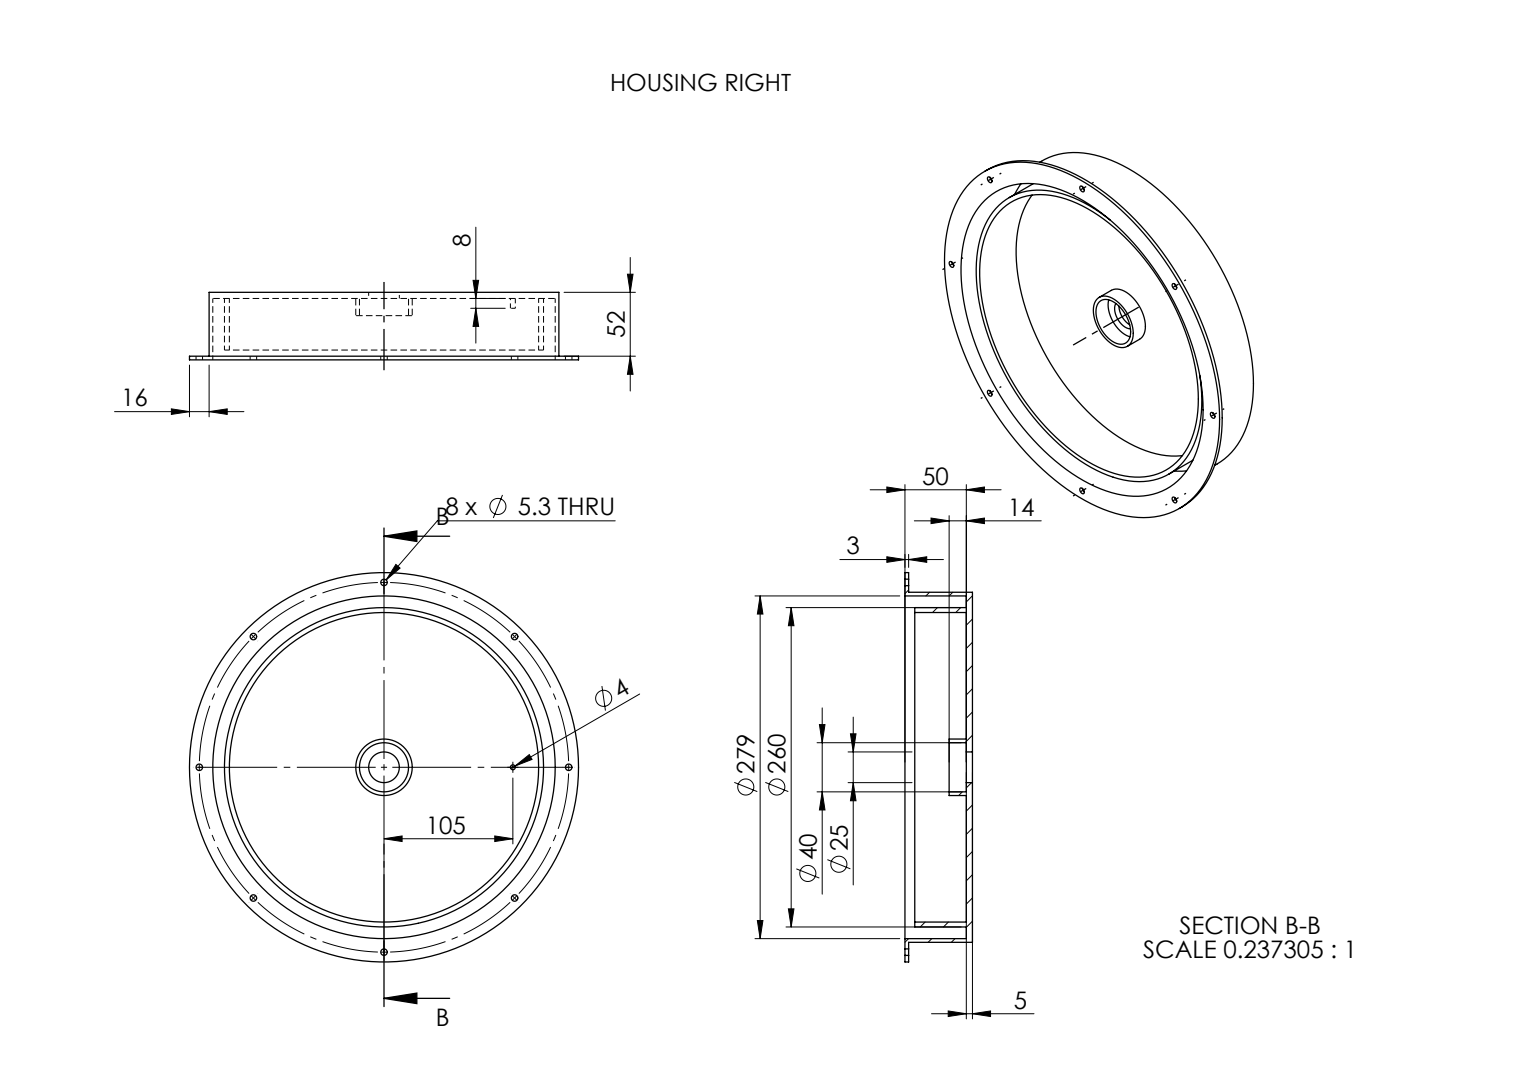
ISO-10303-21;
HEADER;
FILE_DESCRIPTION (('STEP AP214'),
    '1' );
FILE_NAME ('housing right.step',
    '2026-10-08T11:45:07',
    ( '' ),
    ( '' ),
    'SwSTEP 2.0',
    'SolidWorks 2026',
    '' );
FILE_SCHEMA (( 'AUTOMOTIVE_DESIGN' ));
ENDSEC;

DATA;
#35=CIRCLE ( 'NONE', #41130, 12.49999999999993427 ) ;
#48=DIRECTION ( 'NONE',  ( 3.892440008040322386E-16, -2.658563593772947863E-15, -1.000000000000000000 ) ) ;
#71=ORIENTED_EDGE ( 'NONE', *, *, #29230, .F. ) ;
#74=CARTESIAN_POINT ( 'NONE',  ( -3.996523416598931009E-15, 2.658563593772952281E-14, 10.00000000000000178 ) ) ;
#130=EDGE_CURVE ( 'NONE', #29194, #21952, #31734, .T. ) ;
#132=CIRCLE ( 'NONE', #17653, 142.4999999999992610 ) ;
#196=DIRECTION ( 'NONE',  ( -3.996523416598930318E-16, 2.658563593772947863E-15, 1.000000000000000000 ) ) ;
#215=DIRECTION ( 'NONE',  ( 1.000000000000000000, 0.000000000000000000, -3.273063162220425331E-16 ) ) ;
#239=VERTEX_POINT ( 'NONE', #9633 ) ;
#246=CARTESIAN_POINT ( 'NONE',  ( 150.4999999999986926, 1.388241670201576064E-12, 6.999999999999959144 ) ) ;
#281=CARTESIAN_POINT ( 'NONE',  ( 106.9999999999993179, -2.318365118890836037E-13, -32.00000000000000000 ) ) ;
#401=EDGE_CURVE ( 'NONE', #35963, #19047, #6638, .T. ) ;
#561=CIRCLE ( 'NONE', #25023, 12.49999999999993427 ) ;
#699=ORIENTED_EDGE ( 'NONE', *, *, #10056, .T. ) ;
#888=DIRECTION ( 'NONE',  ( 1.000000000000000000, -1.373900992973641868E-15, -3.994789077170585140E-16 ) ) ;
#928=EDGE_CURVE ( 'NONE', #37599, #28601, #37468, .T. ) ;
#942=DIRECTION ( 'NONE',  ( -3.996523416598930318E-16, 2.658563593772947863E-15, 1.000000000000000000 ) ) ;
#955=CARTESIAN_POINT ( 'NONE',  ( -139.4999999999992610, 2.182448244575515701E-13, 10.00000000000005684 ) ) ;
#1042=FACE_BOUND ( 'NONE', #4502, .T. ) ;
#1092=EDGE_LOOP ( 'NONE', ( #29241, #12983 ) ) ;
#1130=AXIS2_PLACEMENT_3D ( 'NONE', #36549, #35909, #36340 ) ;
#1195=CARTESIAN_POINT ( 'NONE',  ( -2.107686228591307694E-13, 150.5000000000013642, 10.00000000000041922 ) ) ;
#1201=CIRCLE ( 'NONE', #28408, 158.4999999999992042 ) ;
#1256=DIRECTION ( 'NONE',  ( -3.996523416598930318E-16, 2.658563593772947863E-15, 1.000000000000000000 ) ) ;
#1258=CARTESIAN_POINT ( 'NONE',  ( -106.4195705685749402, 106.4195705685765745, 7.000000000000337508 ) ) ;
#1259=VECTOR ( 'NONE', #5273, 1000.000000000000000 ) ;
#1261=DIRECTION ( 'NONE',  ( -3.996523416598930318E-16, 2.658563593772947863E-15, 1.000000000000000000 ) ) ;
#1275=PLANE ( 'NONE',  #36174 ) ;
#1282=DIRECTION ( 'NONE',  ( 1.000000000000000000, -1.373900992973641868E-15, -3.994789077170585140E-16 ) ) ;
#1310=DIRECTION ( 'NONE',  ( -3.996523416598930318E-16, 2.658563593772947863E-15, 1.000000000000000000 ) ) ;
#1351=ORIENTED_EDGE ( 'NONE', *, *, #21891, .F. ) ;
#1373=FILL_AREA_STYLE ('',( #25619 ) ) ;
#1422=DIRECTION ( 'NONE',  ( 1.000000000000000000, 0.000000000000000000, -6.546126324440832913E-16 ) ) ;
#1454=CIRCLE ( 'NONE', #18933, 2.649999999999979039 ) ;
#1460=AXIS2_PLACEMENT_3D ( 'NONE', #22396, #26282, #32380 ) ;
#1470=DIRECTION ( 'NONE',  ( 1.000000000000000000, 0.000000000000000000, -6.546126324440850663E-16 ) ) ;
#1495=AXIS2_PLACEMENT_3D ( 'NONE', #18764, #1256, #11313 ) ;
#1513=EDGE_CURVE ( 'NONE', #34370, #34755, #40157, .T. ) ;
#1523=DIRECTION ( 'NONE',  ( -3.996523416598930318E-16, 2.658563593772947863E-15, 1.000000000000000000 ) ) ;
#1539=ADVANCED_FACE ( 'NONE', ( #18278 ), #14551, .T. ) ;
#1612=ORIENTED_EDGE ( 'NONE', *, *, #24949, .T. ) ;
#1654=EDGE_CURVE ( 'NONE', #20992, #25205, #27692, .T. ) ;
#1669=VECTOR ( 'NONE', #942, 1000.000000000000000 ) ;
#1692=LINE ( 'NONE', #4529, #37119 ) ;
#1705=EDGE_CURVE ( 'NONE', #13925, #12177, #32177, .T. ) ;
#1804=SURFACE_STYLE_USAGE ( .BOTH. , #18872 ) ;
#1807=EDGE_LOOP ( 'NONE', ( #11294, #17144 ) ) ;
#1888=AXIS2_PLACEMENT_3D ( 'NONE', #35141, #2178, #24725 ) ;
#2004=EDGE_CURVE ( 'NONE', #41484, #24680, #21070, .T. ) ;
#2042=ORIENTED_EDGE ( 'NONE', *, *, #2004, .T. ) ;
#2045=DIRECTION ( 'NONE',  ( 3.996523416598993920E-16, 2.658563593772947074E-15, 1.000000000000000000 ) ) ;
#2057=EDGE_CURVE ( 'NONE', #25205, #20992, #33192, .T. ) ;
#2087=VECTOR ( 'NONE', #14850, 1000.000000000000000 ) ;
#2101=DIRECTION ( 'NONE',  ( -3.996523416598930318E-16, 2.658563593772947863E-15, 1.000000000000000000 ) ) ;
#2138=DIRECTION ( 'NONE',  ( 3.996523416598930318E-16, -2.658563593772947863E-15, -1.000000000000000000 ) ) ;
#2151=VERTEX_POINT ( 'NONE', #41176 ) ;
#2178=DIRECTION ( 'NONE',  ( -3.996523416598930318E-16, 2.658563593772947863E-15, 1.000000000000000000 ) ) ;
#2190=CARTESIAN_POINT ( 'NONE',  ( 104.9999999999993321, -2.506021480131494702E-13, -40.00000000000000000 ) ) ;
#2216=SURFACE_STYLE_USAGE ( .BOTH. , #5718 ) ;
#2237=DIRECTION ( 'NONE',  ( 3.996523416598930318E-16, -2.658563593772947863E-15, -1.000000000000000000 ) ) ;
#2270=ORIENTED_EDGE ( 'NONE', *, *, #38290, .T. ) ;
#2365=CARTESIAN_POINT ( 'NONE',  ( 23.00000000000001066, -1.165156337948621952E-13, -25.99999999999999289 ) ) ;
#2396=ORIENTED_EDGE ( 'NONE', *, *, #28334, .F. ) ;
#2434=PLANE ( 'NONE',  #33908 ) ;
#2445=CARTESIAN_POINT ( 'NONE',  ( -24.83242019125695421, 113.3108596183312216, 2.000000000000327738 ) ) ;
#2465=EDGE_CURVE ( 'NONE', #28601, #37599, #42175, .T. ) ;
#2478=DIRECTION ( 'NONE',  ( -3.996523416598930318E-16, 2.658563593772947863E-15, 1.000000000000000000 ) ) ;
#2537=AXIS2_PLACEMENT_3D ( 'NONE', #41329, #11482, #24817 ) ;
#2636=CYLINDRICAL_SURFACE ( 'NONE', #18326, 158.4999999999992042 ) ;
#2638=EDGE_CURVE ( 'NONE', #38278, #24835, #38702, .T. ) ;
#2665=DIRECTION ( 'NONE',  ( 1.000000000000000000, -1.373900992973642263E-15, 0.000000000000000000 ) ) ;
#2673=CYLINDRICAL_SURFACE ( 'NONE', #25111, 19.99999999999989342 ) ;
#2692=CYLINDRICAL_SURFACE ( 'NONE', #35754, 2.649999999999979039 ) ;
#2714=EDGE_LOOP ( 'NONE', ( #26003, #5036, #29046, #42550 ) ) ;
#2731=CYLINDRICAL_SURFACE ( 'NONE', #26813, 12.49999999999993427 ) ;
#2791=EDGE_CURVE ( 'NONE', #36354, #9697, #17894, .T. ) ;
#2817=DIRECTION ( 'NONE',  ( 1.000000000000000000, 0.000000000000000000, -3.273063162220416457E-16 ) ) ;
#2847=EDGE_LOOP ( 'NONE', ( #27807, #15265 ) ) ;
#2852=CARTESIAN_POINT ( 'NONE',  ( -139.4999999999999716, 1.517807346132291325E-13, -40.00000000000005684 ) ) ;
#2893=DIRECTION ( 'NONE',  ( -3.996523416598930318E-16, 2.658563593772947863E-15, 1.000000000000000000 ) ) ;
#2967=CARTESIAN_POINT ( 'NONE',  ( -142.5000000000000000, 1.627194001049080943E-13, -45.00000000000004974 ) ) ;
#2977=CARTESIAN_POINT ( 'NONE',  ( 126.0000000000000568, -2.077321393419925476E-13, -39.99999999999992895 ) ) ;
#3020=DIRECTION ( 'NONE',  ( -1.000000000000000000, 1.373900992973641868E-15, 3.469446951953632924E-16 ) ) ;
#3024=ADVANCED_FACE ( 'NONE', ( #26080 ), #9700, .F. ) ;
#3066=FACE_BOUND ( 'NONE', #13828, .T. ) ;
#3120=DIRECTION ( 'NONE',  ( -3.996523416598930318E-16, 2.658563593772947863E-15, 1.000000000000000000 ) ) ;
#3131=DIRECTION ( 'NONE',  ( -3.996523416598930318E-16, 2.658563593772947863E-15, 1.000000000000000000 ) ) ;
#3156=CARTESIAN_POINT ( 'NONE',  ( -19.99999999999998934, -6.025457873503454466E-14, -26.00000000000001066 ) ) ;
#3170=AXIS2_PLACEMENT_3D ( 'NONE', #25052, #18077, #31766 ) ;
#3264=AXIS2_PLACEMENT_3D ( 'NONE', #13667, #24140, #3577 ) ;
#3280=EDGE_LOOP ( 'NONE', ( #4077, #12239, #21262, #32611 ) ) ;
#3329=AXIS2_PLACEMENT_3D ( 'NONE', #11939, #28527, #38091 ) ;
#3410=DIRECTION ( 'NONE',  ( 1.000000000000000000, 0.000000000000000000, -6.546126324440850663E-16 ) ) ;
#3459=ADVANCED_FACE ( 'NONE', ( #5721 ), #35603, .F. ) ;
#3474=DIRECTION ( 'NONE',  ( 1.000000000000000000, -1.373900992973641868E-15, -4.017254365419995317E-16 ) ) ;
#3539=DIRECTION ( 'NONE',  ( -3.996523416598930318E-16, 2.658563593772947863E-15, 1.000000000000000000 ) ) ;
#3549=VERTEX_POINT ( 'NONE', #2852 ) ;
#3577=DIRECTION ( 'NONE',  ( 1.000000000000000000, -1.373900992973642066E-15, -3.854941057726257326E-16 ) ) ;
#3634=ADVANCED_FACE ( 'NONE', ( #29950 ), #24291, .F. ) ;
#3638=EDGE_CURVE ( 'NONE', #11569, #32279, #21241, .T. ) ;
#3662=EDGE_LOOP ( 'NONE', ( #38086, #23873 ) ) ;
#3722=CARTESIAN_POINT ( 'NONE',  ( 147.8499999999987153, 1.396194884625391392E-12, 9.999999999999960920 ) ) ;
#3733=AXIS2_PLACEMENT_3D ( 'NONE', #39429, #9127, #6070 ) ;
#3754=ORIENTED_EDGE ( 'NONE', *, *, #35389, .T. ) ;
#3757=ORIENTED_EDGE ( 'NONE', *, *, #35139, .T. ) ;
#3773=ORIENTED_EDGE ( 'NONE', *, *, #30193, .T. ) ;
#3794=ADVANCED_FACE ( 'NONE', ( #21234 ), #31884, .F. ) ;
#3839=EDGE_LOOP ( 'NONE', ( #23186, #13408 ) ) ;
#3852=CARTESIAN_POINT ( 'NONE',  ( 0.000000000000000000, 0.000000000000000000, 0.000000000000000000 ) ) ;
#3970=VECTOR ( 'NONE', #21919, 1000.000000000000000 ) ;
#4011=CARTESIAN_POINT ( 'NONE',  ( 106.4195705685734623, 106.4195705685780524, 10.00000000000025402 ) ) ;
#4044=AXIS2_PLACEMENT_3D ( 'NONE', #5844, #28374, #14845 ) ;
#4077=ORIENTED_EDGE ( 'NONE', *, *, #40367, .F. ) ;
#4086=ADVANCED_FACE ( 'NONE', ( #31583 ), #28757, .F. ) ;
#4136=ORIENTED_EDGE ( 'NONE', *, *, #8514, .T. ) ;
#4160=ADVANCED_BREP_SHAPE_REPRESENTATION ( '', ( #13589, #13552 ), #31631 ) ;
#4180=DIRECTION ( 'NONE',  ( -3.996523416598930318E-16, 2.658563593772947863E-15, 1.000000000000000000 ) ) ;
#4181=EDGE_LOOP ( 'NONE', ( #12378, #30826, #3773, #26628 ) ) ;
#4221=FACE_BOUND ( 'NONE', #10756, .T. ) ;
#4254=ORIENTED_EDGE ( 'NONE', *, *, #1513, .T. ) ;
#4297=DIRECTION ( 'NONE',  ( -3.996523416598930318E-16, 2.658563593772947863E-15, 1.000000000000000000 ) ) ;
#4303=DIRECTION ( 'NONE',  ( -3.996523416598930318E-16, 2.658563593772947863E-15, 1.000000000000000000 ) ) ;
#4332=ORIENTED_EDGE ( 'NONE', *, *, #24391, .F. ) ;
#4344=VERTEX_POINT ( 'NONE', #7599 ) ;
#4367=ORIENTED_EDGE ( 'NONE', *, *, #36129, .F. ) ;
#4368=CARTESIAN_POINT ( 'NONE',  ( -109.0695705685749317, 106.4195705685765603, 10.00000000000033573 ) ) ;
#4438=CARTESIAN_POINT ( 'NONE',  ( 1.598609366639573350E-14, -1.063425437509180407E-13, -40.00000000000000000 ) ) ;
#4449=AXIS2_PLACEMENT_3D ( 'NONE', #40376, #7006, #20157 ) ;
#4454=ORIENTED_EDGE ( 'NONE', *, *, #7875, .F. ) ;
#4488=DIRECTION ( 'NONE',  ( -3.996523416598930318E-16, 2.658563593772947863E-15, 1.000000000000000000 ) ) ;
#4502=EDGE_LOOP ( 'NONE', ( #15982, #4454 ) ) ;
#4513=DIRECTION ( 'NONE',  ( -1.000000000000000000, 1.373900992973642066E-15, 3.979293995072266947E-16 ) ) ;
#4529=CARTESIAN_POINT ( 'NONE',  ( 109.0695705685756565, -106.4195705685758213, 9.999999999999667821 ) ) ;
#4583=EDGE_LOOP ( 'NONE', ( #30063, #12227 ) ) ;
#4597=CARTESIAN_POINT ( 'NONE',  ( -109.0695705685741785, -106.4195705685773135, 6.999999999999753975 ) ) ;
#4724=VECTOR ( 'NONE', #10466, 1000.000000000000000 ) ;
#4732=DIRECTION ( 'NONE',  ( 1.000000000000000000, 0.000000000000000000, -6.546126324440832913E-16 ) ) ;
#4747=DIRECTION ( 'NONE',  ( -3.996523416598930318E-16, 2.658563593772947863E-15, 1.000000000000000000 ) ) ;
#4775=VECTOR ( 'NONE', #27728, 1000.000000000000000 ) ;
#4776=FACE_BOUND ( 'NONE', #41078, .T. ) ;
#4870=( NAMED_UNIT ( * ) SI_UNIT ( $, .STERADIAN. ) SOLID_ANGLE_UNIT ( ) );
#4942=CARTESIAN_POINT ( 'NONE',  ( 1.798435537469519230E-14, -1.196353617197826191E-13, -44.99999999999999289 ) ) ;
#4970=DIRECTION ( 'NONE',  ( 1.000000000000000000, -1.373900992973642066E-15, -3.979293995072266947E-16 ) ) ;
#4973=CIRCLE ( 'NONE', #7043, 2.649999999999973266 ) ;
#5036=ORIENTED_EDGE ( 'NONE', *, *, #1654, .F. ) ;
#5038=DIRECTION ( 'NONE',  ( -3.996523416598930318E-16, 2.658563593772947863E-15, 1.000000000000000000 ) ) ;
#5113=FACE_BOUND ( 'NONE', #4583, .T. ) ;
#5117=VERTEX_POINT ( 'NONE', #25453 ) ;
#5125=DIRECTION ( 'NONE',  ( 1.000000000000000000, 0.000000000000000000, -3.273063162220416457E-16 ) ) ;
#5129=CIRCLE ( 'NONE', #23286, 2.649999999999957723 ) ;
#5147=EDGE_CURVE ( 'NONE', #34755, #34370, #1454, .T. ) ;
#5259=AXIS2_PLACEMENT_3D ( 'NONE', #8434, #21998, #4732 ) ;
#5273=DIRECTION ( 'NONE',  ( -3.996523416598930318E-16, 2.658563593772947863E-15, 1.000000000000000000 ) ) ;
#5304=CIRCLE ( 'NONE', #6656, 125.9999999999993605 ) ;
#5453=AXIS2_PLACEMENT_3D ( 'NONE', #39950, #22798, #39534 ) ;
#5480=CARTESIAN_POINT ( 'NONE',  ( 1.598609366639573350E-14, -1.063425437509180407E-13, -40.00000000000000000 ) ) ;
#5595=CARTESIAN_POINT ( 'NONE',  ( -103.7695705685749772, 106.4195705685765745, 10.00000000000033396 ) ) ;
#5623=ORIENTED_EDGE ( 'NONE', *, *, #10507, .F. ) ;
#5650=AXIS2_PLACEMENT_3D ( 'NONE', #27391, #20437, #13666 ) ;
#5678=ORIENTED_EDGE ( 'NONE', *, *, #24651, .T. ) ;
#5693=ORIENTED_EDGE ( 'NONE', *, *, #25641, .F. ) ;
#5714=DIRECTION ( 'NONE',  ( -3.996523416598930318E-16, 2.658563593772947863E-15, 1.000000000000000000 ) ) ;
#5718=SURFACE_SIDE_STYLE ('',( #38885 ) ) ;
#5721=FACE_OUTER_BOUND ( 'NONE', #3280, .T. ) ;
#5724=ORIENTED_EDGE ( 'NONE', *, *, #35189, .T. ) ;
#5740=ORIENTED_EDGE ( 'NONE', *, *, #21265, .T. ) ;
#5743=CYLINDRICAL_SURFACE ( 'NONE', #28436, 2.649999999999971934 ) ;
#5782=CYLINDRICAL_SURFACE ( 'NONE', #3329, 12.49999999999993427 ) ;
#5803=ORIENTED_EDGE ( 'NONE', *, *, #37006, .T. ) ;
#5818=CIRCLE ( 'NONE', #29501, 19.99999999999989342 ) ;
#5844=CARTESIAN_POINT ( 'NONE',  ( -106.4195705685749402, 106.4195705685765745, 10.00000000000033573 ) ) ;
#5846=AXIS2_PLACEMENT_3D ( 'NONE', #24235, #10672, #33575 ) ;
#5854=ORIENTED_EDGE ( 'NONE', *, *, #928, .T. ) ;
#5921=CARTESIAN_POINT ( 'NONE',  ( 1.039096088315723056E-14, -6.912265343809663812E-14, -26.00000000000000355 ) ) ;
#5922=AXIS2_PLACEMENT_3D ( 'NONE', #1195, #41554, #11702 ) ;
#5942=DIRECTION ( 'NONE',  ( -3.996523416598930318E-16, 2.658563593772947863E-15, 1.000000000000000000 ) ) ;
#5971=AXIS2_PLACEMENT_3D ( 'NONE', #27064, #34441, #1282 ) ;
#6033=DIRECTION ( 'NONE',  ( 1.000000000000000000, -1.373900992973641277E-15, -5.551115123125812284E-16 ) ) ;
#6070=DIRECTION ( 'NONE',  ( 1.000000000000000000, 0.000000000000000000, -3.273063162220425331E-16 ) ) ;
#6101=AXIS2_PLACEMENT_3D ( 'NONE', #2445, #15809, #42388 ) ;
#6122=CIRCLE ( 'NONE', #10304, 19.99999999999989342 ) ;
#6221=CARTESIAN_POINT ( 'NONE',  ( 139.5000000000000284, -2.144538195783110118E-13, -39.99999999999994316 ) ) ;
#6239=DIRECTION ( 'NONE',  ( -3.996523416598930318E-16, 2.658563593772947863E-15, 1.000000000000000000 ) ) ;
#6244=VERTEX_POINT ( 'NONE', #26614 ) ;
#6245=CARTESIAN_POINT ( 'NONE',  ( 1.798435537469519230E-14, -1.196353617197826191E-13, -44.99999999999999289 ) ) ;
#6312=ADVANCED_FACE ( 'NONE', ( #24231, #17911, #20746, #31186, #4776, #30544, #1042, #34655, #27473, #37497 ), #1275, .T. ) ;
#6331=FACE_OUTER_BOUND ( 'NONE', #38808, .T. ) ;
#6413=DIRECTION ( 'NONE',  ( 3.996523416598930318E-16, -2.658563593772947863E-15, -1.000000000000000000 ) ) ;
#6414=CIRCLE ( 'NONE', #30821, 125.9999999999993605 ) ;
#6445=DIRECTION ( 'NONE',  ( -3.996523416598930318E-16, 2.658563593772947863E-15, 1.000000000000000000 ) ) ;
#6505=STYLED_ITEM ( 'NONE', ( #31931 ), #4160 ) ;
#6638=CIRCLE ( 'NONE', #12249, 158.4999999999992042 ) ;
#6650=DIRECTION ( 'NONE',  ( 1.000000000000000000, 0.000000000000000000, -6.546126324440850663E-16 ) ) ;
#6656=AXIS2_PLACEMENT_3D ( 'NONE', #24085, #30618, #37573 ) ;
#6696=ORIENTED_EDGE ( 'NONE', *, *, #33011, .F. ) ;
#6721=AXIS2_PLACEMENT_3D ( 'NONE', #39446, #9352, #9581 ) ;
#6826=CYLINDRICAL_SURFACE ( 'NONE', #23976, 2.649999999999979039 ) ;
#6875=CYLINDRICAL_SURFACE ( 'NONE', #5650, 129.9999999999993463 ) ;
#6926=CARTESIAN_POINT ( 'NONE',  ( -150.4999999999986926, -2.921102061156358310E-13, 10.00000000000004441 ) ) ;
#6938=FACE_OUTER_BOUND ( 'NONE', #28430, .T. ) ;
#6992=DIRECTION ( 'NONE',  ( 1.000000000000000000, 0.000000000000000000, -6.546126324440850663E-16 ) ) ;
#7001=ORIENTED_EDGE ( 'NONE', *, *, #12745, .T. ) ;
#7004=CIRCLE ( 'NONE', #41129, 2.649999999999971934 ) ;
#7006=DIRECTION ( 'NONE',  ( -3.996523416598930318E-16, 2.658563593772947863E-15, 1.000000000000000000 ) ) ;
#7038=ORIENTED_EDGE ( 'NONE', *, *, #33624, .T. ) ;
#7039=AXIS2_PLACEMENT_3D ( 'NONE', #8455, #21605, #15266 ) ;
#7043=AXIS2_PLACEMENT_3D ( 'NONE', #13886, #33052, #27182 ) ;
#7081=DIRECTION ( 'NONE',  ( -3.996523416598930318E-16, 2.658563593772947863E-15, 1.000000000000000000 ) ) ;
#7134=ORIENTED_EDGE ( 'NONE', *, *, #39605, .F. ) ;
#7188=VERTEX_POINT ( 'NONE', #4597 ) ;
#7241=DIRECTION ( 'NONE',  ( 3.996523416598930318E-16, -2.658563593772947863E-15, -1.000000000000000000 ) ) ;
#7243=CARTESIAN_POINT ( 'NONE',  ( -19.99999999999998224, -6.025457873503436795E-14, -40.00000000000000711 ) ) ;
#7277=CARTESIAN_POINT ( 'NONE',  ( 1.598609366639573350E-14, -1.063425437509180407E-13, -40.00000000000000000 ) ) ;
#7296=DIRECTION ( 'NONE',  ( -3.996523416598930318E-16, 2.658563593772947863E-15, 1.000000000000000000 ) ) ;
#7301=ORIENTED_EDGE ( 'NONE', *, *, #40139, .F. ) ;
#7463=EDGE_LOOP ( 'NONE', ( #17351, #12263, #14343, #4367 ) ) ;
#7512=DIRECTION ( 'NONE',  ( 3.996523416598930318E-16, -2.658563593772947863E-15, -1.000000000000000000 ) ) ;
#7517=CARTESIAN_POINT ( 'NONE',  ( -103.7695705685742240, -106.4195705685773135, 9.999999999999751310 ) ) ;
#7578=EDGE_CURVE ( 'NONE', #7188, #43139, #14414, .T. ) ;
#7588=AXIS2_PLACEMENT_3D ( 'NONE', #22582, #15593, #28897 ) ;
#7599=CARTESIAN_POINT ( 'NONE',  ( -126.0000000000000284, 1.230603612181078346E-13, 1.999999999999952704 ) ) ;
#7651=EDGE_CURVE ( 'NONE', #22603, #21952, #28587, .T. ) ;
#7692=CARTESIAN_POINT ( 'NONE',  ( 1.798435537469519230E-14, -1.196353617197826191E-13, -44.99999999999999289 ) ) ;
#7695=CARTESIAN_POINT ( 'NONE',  ( 106.9999999999993321, -2.424707662641753068E-13, -40.00000000000000000 ) ) ;
#7718=ADVANCED_FACE ( 'NONE', ( #31204 ), #41858, .F. ) ;
#7741=DIRECTION ( 'NONE',  ( 1.000000000000000000, -1.373900992973642263E-15, -3.736327486719295592E-16 ) ) ;
#7809=DIRECTION ( 'NONE',  ( -3.996523416598930318E-16, 2.658563593772947863E-15, 1.000000000000000000 ) ) ;
#7818=ORIENTED_EDGE ( 'NONE', *, *, #12311, .T. ) ;
#7836=ORIENTED_EDGE ( 'NONE', *, *, #9323, .F. ) ;
#7875=EDGE_CURVE ( 'NONE', #42975, #29643, #20300, .T. ) ;
#7923=ADVANCED_FACE ( 'NONE', ( #29431, #26156, #25539 ), #39431, .T. ) ;
#7932=ORIENTED_EDGE ( 'NONE', *, *, #19309, .T. ) ;
#7977=CYLINDRICAL_SURFACE ( 'NONE', #13481, 2.649999999999979039 ) ;
#8063=CARTESIAN_POINT ( 'NONE',  ( -109.0695705685749317, 106.4195705685765603, 7.000000000000336620 ) ) ;
#8203=ORIENTED_EDGE ( 'NONE', *, *, #23450, .F. ) ;
#8284=CIRCLE ( 'NONE', #31276, 130.0000000000013927 ) ;
#8285=ORIENTED_EDGE ( 'NONE', *, *, #26316, .F. ) ;
#8329=ORIENTED_EDGE ( 'NONE', *, *, #35389, .F. ) ;
#8423=ADVANCED_FACE ( 'NONE', ( #17167 ), #6875, .T. ) ;
#8434=CARTESIAN_POINT ( 'NONE',  ( 2.027755760259328333E-13, -150.5000000000013642, 9.999999999999586109 ) ) ;
#8455=CARTESIAN_POINT ( 'NONE',  ( 104.9999999999993321, -2.293336392629658115E-13, -32.00000000000000000 ) ) ;
#8514=EDGE_CURVE ( 'NONE', #21952, #29194, #4973, .T. ) ;
#8531=DIRECTION ( 'NONE',  ( 1.000000000000000000, -1.373900992973642066E-15, -3.854941057726257326E-16 ) ) ;
#8539=EDGE_LOOP ( 'NONE', ( #27289, #22347, #21596, #18498 ) ) ;
#8607=EDGE_CURVE ( 'NONE', #29204, #43139, #14059, .T. ) ;
#8658=DIRECTION ( 'NONE',  ( 3.996523416598930318E-16, -2.658563593772947863E-15, -1.000000000000000000 ) ) ;
#8698=CARTESIAN_POINT ( 'NONE',  ( 2.649999999999768541, 150.5000000000013642, 10.00000000000041567 ) ) ;
#8724=VERTEX_POINT ( 'NONE', #19900 ) ;
#8768=VECTOR ( 'NONE', #2893, 1000.000000000000000 ) ;
#8786=( NAMED_UNIT ( * ) PLANE_ANGLE_UNIT ( ) SI_UNIT ( $, .RADIAN. ) );
#8921=FACE_OUTER_BOUND ( 'NONE', #36499, .T. ) ;
#9017=CARTESIAN_POINT ( 'NONE',  ( 1.598609366639573350E-14, -1.063425437509180407E-13, -40.00000000000000000 ) ) ;
#9023=PLANE ( 'NONE',  #6101 ) ;
#9026=SHAPE_REPRESENTATION ( 'housing right', ( #13552 ), #31631 ) ;
#9076=CARTESIAN_POINT ( 'NONE',  ( 2.649999999999769873, 150.5000000000013642, 7.000000000000418332 ) ) ;
#9088=CARTESIAN_POINT ( 'NONE',  ( 129.9999999999992042, 8.206338904687194424E-13, 369.6955262170047263 ) ) ;
#9127=DIRECTION ( 'NONE',  ( -3.996523416598930318E-16, 2.658563593772947863E-15, 1.000000000000000000 ) ) ;
#9132=LINE ( 'NONE', #15708, #23630 ) ;
#9154=VERTEX_POINT ( 'NONE', #8063 ) ;
#9219=ORIENTED_EDGE ( 'NONE', *, *, #20013, .T. ) ;
#9323=EDGE_CURVE ( 'NONE', #37475, #5117, #132, .T. ) ;
#9352=DIRECTION ( 'NONE',  ( 3.996523416598930318E-16, -2.658563593772947863E-15, -1.000000000000000000 ) ) ;
#9359=ORIENTED_EDGE ( 'NONE', *, *, #31108, .F. ) ;
#9525=ORIENTED_EDGE ( 'NONE', *, *, #1654, .T. ) ;
#9565=ORIENTED_EDGE ( 'NONE', *, *, #20142, .F. ) ;
#9581=DIRECTION ( 'NONE',  ( -1.000000000000000000, 1.373900992973642066E-15, 4.525365589504737954E-16 ) ) ;
#9604=ORIENTED_EDGE ( 'NONE', *, *, #33858, .F. ) ;
#9633=CARTESIAN_POINT ( 'NONE',  ( 130.0000000000000568, -2.127378845942283338E-13, -39.99999999999995026 ) ) ;
#9681=ORIENTED_EDGE ( 'NONE', *, *, #26998, .F. ) ;
#9697=VERTEX_POINT ( 'NONE', #16524 ) ;
#9700=CYLINDRICAL_SURFACE ( 'NONE', #12217, 125.9999999999993605 ) ;
#9745=ORIENTED_EDGE ( 'NONE', *, *, #3638, .T. ) ;
#9749=EDGE_CURVE ( 'NONE', #26054, #42401, #12804, .T. ) ;
#9767=EDGE_CURVE ( 'NONE', #34370, #21317, #15659, .T. ) ;
#9776=CYLINDRICAL_SURFACE ( 'NONE', #37511, 2.649999999999957723 ) ;
#9828=EDGE_CURVE ( 'NONE', #9154, #6244, #26524, .T. ) ;
#9831=CARTESIAN_POINT ( 'NONE',  ( 142.4999999999992610, -1.771709463423323217E-13, 6.999999999999945821 ) ) ;
#9873=VECTOR ( 'NONE', #33300, 1000.000000000000000 ) ;
#9919=CYLINDRICAL_SURFACE ( 'NONE', #41503, 158.4999999999992042 ) ;
#10056=EDGE_CURVE ( 'NONE', #22786, #24835, #17828, .T. ) ;
#10082=DIRECTION ( 'NONE',  ( -3.996523416598930318E-16, 2.658563593772947863E-15, 1.000000000000000000 ) ) ;
#10133=AXIS2_PLACEMENT_3D ( 'NONE', #35928, #42902, #42262 ) ;
#10137=DIRECTION ( 'NONE',  ( 1.000000000000000000, -1.373900992973641868E-15, -4.049512215214018063E-16 ) ) ;
#10148=CARTESIAN_POINT ( 'NONE',  ( 103.7695705685734850, 106.4195705685780524, 10.00000000000025402 ) ) ;
#10213=DIRECTION ( 'NONE',  ( 1.000000000000000000, 0.000000000000000000, 0.000000000000000000 ) ) ;
#10245=VECTOR ( 'NONE', #3131, 1000.000000000000000 ) ;
#10271=AXIS2_PLACEMENT_3D ( 'NONE', #31318, #31742, #24801 ) ;
#10276=AXIS2_PLACEMENT_3D ( 'NONE', #15594, #2237, #26264 ) ;
#10304=AXIS2_PLACEMENT_3D ( 'NONE', #4438, #30868, #37610 ) ;
#10347=ORIENTED_EDGE ( 'NONE', *, *, #33012, .T. ) ;
#10381=CARTESIAN_POINT ( 'NONE',  ( -106.4195705685749402, 106.4195705685765745, 7.000000000000337508 ) ) ;
#10387=CARTESIAN_POINT ( 'NONE',  ( 22.99999999999988987, -9.790568863845134872E-14, -26.00000000000001421 ) ) ;
#10412=DIRECTION ( 'NONE',  ( -3.996523416598930318E-16, 2.658563593772947863E-15, 1.000000000000000000 ) ) ;
#10466=DIRECTION ( 'NONE',  ( 3.996523416598930318E-16, -2.658563593772947863E-15, -1.000000000000000000 ) ) ;
#10471=ORIENTED_EDGE ( 'NONE', *, *, #33011, .T. ) ;
#10486=ORIENTED_EDGE ( 'NONE', *, *, #32018, .F. ) ;
#10492=CARTESIAN_POINT ( 'NONE',  ( -2.797566391619251075E-15, 1.860994515641065082E-14, 7.000000000000002665 ) ) ;
#10507=EDGE_CURVE ( 'NONE', #26054, #25656, #35, .T. ) ;
#10510=AXIS2_PLACEMENT_3D ( 'NONE', #25918, #12398, #4970 ) ;
#10571=CIRCLE ( 'NONE', #1495, 19.99999999999989342 ) ;
#10572=EDGE_LOOP ( 'NONE', ( #20458, #14340 ) ) ;
#10596=ORIENTED_EDGE ( 'NONE', *, *, #7578, .T. ) ;
#10599=CYLINDRICAL_SURFACE ( 'NONE', #24593, 2.649999999999971934 ) ;
#10672=DIRECTION ( 'NONE',  ( -3.996523416598930318E-16, 2.658563593772947863E-15, 1.000000000000000000 ) ) ;
#10752=CARTESIAN_POINT ( 'NONE',  ( -106.4195705685749402, 106.4195705685765745, 10.00000000000033751 ) ) ;
#10756=EDGE_LOOP ( 'NONE', ( #16511, #16642 ) ) ;
#10848=EDGE_CURVE ( 'NONE', #18098, #23944, #25889, .T. ) ;
#10875=ADVANCED_FACE ( 'NONE', ( #31587 ), #21387, .F. ) ;
#10877=CIRCLE ( 'NONE', #42885, 2.649999999999971934 ) ;
#10880=LINE ( 'NONE', #41159, #33707 ) ;
#10889=CARTESIAN_POINT ( 'NONE',  ( 104.9999999999993321, -2.506021480131494702E-13, -40.00000000000000000 ) ) ;
#10929=EDGE_CURVE ( 'NONE', #11054, #32971, #10571, .T. ) ;
#10961=AXIS2_PLACEMENT_3D ( 'NONE', #19121, #32386, #12764 ) ;
#10969=AXIS2_PLACEMENT_3D ( 'NONE', #4011, #7081, #6650 ) ;
#11054=VERTEX_POINT ( 'NONE', #3156 ) ;
#11111=ORIENTED_EDGE ( 'NONE', *, *, #30468, .T. ) ;
#11126=ORIENTED_EDGE ( 'NONE', *, *, #10929, .F. ) ;
#11146=ORIENTED_EDGE ( 'NONE', *, *, #30193, .F. ) ;
#11234=FACE_BOUND ( 'NONE', #34698, .T. ) ;
#11236=EDGE_CURVE ( 'NONE', #25205, #8724, #40256, .T. ) ;
#11240=CARTESIAN_POINT ( 'NONE',  ( 158.4999999999992042, -1.991533622299105221E-13, 6.999999999999939604 ) ) ;
#11294=ORIENTED_EDGE ( 'NONE', *, *, #28181, .F. ) ;
#11295=ADVANCED_FACE ( 'NONE', ( #13899 ), #10599, .F. ) ;
#11313=DIRECTION ( 'NONE',  ( 1.000000000000000000, -1.373900992973641868E-15, -3.469446951953632924E-16 ) ) ;
#11323=LINE ( 'NONE', #31597, #42679 ) ;
#11352=EDGE_LOOP ( 'NONE', ( #19713, #16182, #5724, #3757 ) ) ;
#11356=CARTESIAN_POINT ( 'NONE',  ( 103.7695705685734708, 106.4195705685780382, 7.000000000000249578 ) ) ;
#11444=VECTOR ( 'NONE', #7512, 1000.000000000000000 ) ;
#11482=DIRECTION ( 'NONE',  ( 3.996523416598993920E-16, 2.658563593772947074E-15, 1.000000000000000000 ) ) ;
#11509=CYLINDRICAL_SURFACE ( 'NONE', #5259, 2.649999999999979039 ) ;
#11549=CARTESIAN_POINT ( 'NONE',  ( 158.4999999999992042, -1.911776714485916438E-13, 9.999999999999937828 ) ) ;
#11559=CARTESIAN_POINT ( 'NONE',  ( -22.99999999999986855, -3.752293059970304436E-14, -25.99999999999999289 ) ) ;
#11569=VERTEX_POINT ( 'NONE', #27780 ) ;
#11591=CARTESIAN_POINT ( 'NONE',  ( -22.99999999999998224, -5.613287575611343012E-14, -40.00000000000000711 ) ) ;
#11610=CARTESIAN_POINT ( 'NONE',  ( 1.598609366639573350E-14, -1.063425437509180407E-13, -40.00000000000000000 ) ) ;
#11645=EDGE_CURVE ( 'NONE', #38954, #20249, #6414, .T. ) ;
#11678=FACE_OUTER_BOUND ( 'NONE', #41878, .T. ) ;
#11680=EDGE_LOOP ( 'NONE', ( #39097, #16467 ) ) ;
#11702=DIRECTION ( 'NONE',  ( 1.000000000000000000, 0.000000000000000000, -6.546126324440847704E-16 ) ) ;
#11738=ORIENTED_EDGE ( 'NONE', *, *, #33064, .F. ) ;
#11765=AXIS2_PLACEMENT_3D ( 'NONE', #2190, #22116, #39258 ) ;
#11783=ORIENTED_EDGE ( 'NONE', *, *, #32018, .T. ) ;
#11803=ADVANCED_FACE ( 'NONE', ( #15695 ), #19412, .F. ) ;
#11873=SURFACE_STYLE_FILL_AREA ( #42363 ) ;
#11884=EDGE_LOOP ( 'NONE', ( #10486, #41054, #2042, #11111 ) ) ;
#11888=DIRECTION ( 'NONE',  ( 1.000000000000000000, -1.373900992973642263E-15, -3.996523416598957436E-16 ) ) ;
#11939=CARTESIAN_POINT ( 'NONE',  ( 1.798435537469519230E-14, -1.196353617197826191E-13, -44.99999999999999289 ) ) ;
#11944=FACE_OUTER_BOUND ( 'NONE', #7463, .T. ) ;
#11983=ADVANCED_FACE ( 'NONE', ( #11944 ), #34386, .T. ) ;
#12026=CARTESIAN_POINT ( 'NONE',  ( 126.0000000000000284, -2.077321393419931030E-13, 2.000000000000050626 ) ) ;
#12049=CARTESIAN_POINT ( 'NONE',  ( 109.0695705685756565, -106.4195705685758213, 9.999999999999669598 ) ) ;
#12065=ORIENTED_EDGE ( 'NONE', *, *, #21246, .F. ) ;
#12151=PRODUCT_DEFINITION_FORMATION_WITH_SPECIFIED_SOURCE ( 'ANY', '', #29058, .NOT_KNOWN. ) ;
#12167=DIRECTION ( 'NONE',  ( -3.996523416598930318E-16, 2.658563593772947863E-15, 1.000000000000000000 ) ) ;
#12174=FACE_OUTER_BOUND ( 'NONE', #35184, .T. ) ;
#12177=VERTEX_POINT ( 'NONE', #6221 ) ;
#12217=AXIS2_PLACEMENT_3D ( 'NONE', #39344, #6413, #33028 ) ;
#12227=ORIENTED_EDGE ( 'NONE', *, *, #33408, .T. ) ;
#12239=ORIENTED_EDGE ( 'NONE', *, *, #37006, .F. ) ;
#12249=AXIS2_PLACEMENT_3D ( 'NONE', #10492, #1310, #37096 ) ;
#12263=ORIENTED_EDGE ( 'NONE', *, *, #2465, .T. ) ;
#12292=AXIS2_PLACEMENT_3D ( 'NONE', #34264, #27521, #27306 ) ;
#12311=EDGE_CURVE ( 'NONE', #18098, #39874, #13226, .T. ) ;
#12378=ORIENTED_EDGE ( 'NONE', *, *, #24651, .F. ) ;
#12398=DIRECTION ( 'NONE',  ( -3.996523416598930318E-16, 2.658563593772947863E-15, 1.000000000000000000 ) ) ;
#12434=ADVANCED_FACE ( 'NONE', ( #31724, #11234, #18458, #15179, #4221, #25015, #31515, #21941, #28485, #11678 ), #14955, .F. ) ;
#12439=EDGE_CURVE ( 'NONE', #20683, #38278, #17593, .T. ) ;
#12623=DIRECTION ( 'NONE',  ( 1.000000000000000000, -1.373900992973642066E-15, -3.979293995072266947E-16 ) ) ;
#12659=EDGE_CURVE ( 'NONE', #32464, #42401, #35848, .T. ) ;
#12672=AXIS2_PLACEMENT_3D ( 'NONE', #32023, #2101, #28559 ) ;
#12698=DIRECTION ( 'NONE',  ( 1.000000000000000000, -1.373900992973642263E-15, -4.095874873834148624E-16 ) ) ;
#12745=EDGE_CURVE ( 'NONE', #27398, #29194, #33217, .T. ) ;
#12764=DIRECTION ( 'NONE',  ( 1.000000000000000000, -1.373900992973642263E-15, -4.525365589504737954E-16 ) ) ;
#12804=LINE ( 'NONE', #35686, #33635 ) ;
#12856=ORIENTED_EDGE ( 'NONE', *, *, #7578, .F. ) ;
#12900=CYLINDRICAL_SURFACE ( 'NONE', #18032, 1.999999999999988010 ) ;
#12919=ORIENTED_EDGE ( 'NONE', *, *, #25649, .F. ) ;
#12983=ORIENTED_EDGE ( 'NONE', *, *, #36129, .T. ) ;
#13038=DIRECTION ( 'NONE',  ( -3.996523416598930318E-16, 2.658563593772947863E-15, 1.000000000000000000 ) ) ;
#13082=CARTESIAN_POINT ( 'NONE',  ( 1.598609366639573350E-14, -1.063425437509180407E-13, -40.00000000000000000 ) ) ;
#13147=DIRECTION ( 'NONE',  ( -3.996523416598930318E-16, 2.658563593772947863E-15, 1.000000000000000000 ) ) ;
#13192=FACE_OUTER_BOUND ( 'NONE', #25773, .T. ) ;
#13211=AXIS2_PLACEMENT_3D ( 'NONE', #246, #27348, #23877 ) ;
#13226=LINE ( 'NONE', #281, #11444 ) ;
#13325=ADVANCED_FACE ( 'NONE', ( #41359 ), #11509, .F. ) ;
#13384=DIRECTION ( 'NONE',  ( -3.996523416598930318E-16, 2.658563593772947863E-15, 1.000000000000000000 ) ) ;
#13387=DIRECTION ( 'NONE',  ( 1.000000000000000000, -1.373900992973642263E-15, -3.736327486719295592E-16 ) ) ;
#13408=ORIENTED_EDGE ( 'NONE', *, *, #130, .F. ) ;
#13411=PRODUCT_DEFINITION_SHAPE ( 'NONE', 'NONE',  #23650 ) ;
#13481=AXIS2_PLACEMENT_3D ( 'NONE', #31340, #21568, #1422 ) ;
#13492=ORIENTED_EDGE ( 'NONE', *, *, #14242, .F. ) ;
#13552=AXIS2_PLACEMENT_3D ( 'NONE', #3852, #14597, #10213 ) ;
#13589=MANIFOLD_SOLID_BREP ( 'Boss-Extrude1', #35804 ) ;
#13603=ORIENTED_EDGE ( 'NONE', *, *, #26144, .F. ) ;
#13606=CARTESIAN_POINT ( 'NONE',  ( 147.8499999999987153, 1.396194884625391392E-12, 6.999999999999958256 ) ) ;
#13666=DIRECTION ( 'NONE',  ( -1.000000000000000000, 1.373900992973641671E-15, 4.270088556250623393E-16 ) ) ;
#13667=CARTESIAN_POINT ( 'NONE',  ( 2.164352920501968783E-14, -1.058809993658035131E-13, -39.99999999999997868 ) ) ;
#13696=CIRCLE ( 'NONE', #12292, 2.649999999999971934 ) ;
#13795=ADVANCED_FACE ( 'NONE', ( #25214, #24780 ), #28039, .T. ) ;
#13828=EDGE_LOOP ( 'NONE', ( #11126, #8285 ) ) ;
#13835=CARTESIAN_POINT ( 'NONE',  ( 125.9999999999992184, 8.256396357209550266E-13, 369.6955262170047263 ) ) ;
#13858=CIRCLE ( 'NONE', #5453, 2.649999999999971934 ) ;
#13886=CARTESIAN_POINT ( 'NONE',  ( -2.107686228591307694E-13, 150.5000000000013642, 10.00000000000041922 ) ) ;
#13899=FACE_OUTER_BOUND ( 'NONE', #30778, .T. ) ;
#13925=VERTEX_POINT ( 'NONE', #38675 ) ;
#14009=ADVANCED_FACE ( 'NONE', ( #19509, #3066 ), #2434, .T. ) ;
#14054=EDGE_LOOP ( 'NONE', ( #38887, #21103 ) ) ;
#14059=CIRCLE ( 'NONE', #38410, 2.649999999999971934 ) ;
#14188=CARTESIAN_POINT ( 'NONE',  ( -2.650000000000189981, 150.5000000000013642, 10.00000000000041922 ) ) ;
#14216=ORIENTED_EDGE ( 'NONE', *, *, #15129, .T. ) ;
#14226=AXIS2_PLACEMENT_3D ( 'NONE', #24463, #17701, #31847 ) ;
#14242=EDGE_CURVE ( 'NONE', #29604, #17574, #19340, .T. ) ;
#14247=CARTESIAN_POINT ( 'NONE',  ( -103.7695705685749772, 106.4195705685765745, 10.00000000000033573 ) ) ;
#14258=VERTEX_POINT ( 'NONE', #12049 ) ;
#14270=EDGE_CURVE ( 'NONE', #25091, #8724, #35308, .T. ) ;
#14297=DIRECTION ( 'NONE',  ( -3.996523416598930318E-16, 2.658563593772947863E-15, 1.000000000000000000 ) ) ;
#14308=CARTESIAN_POINT ( 'NONE',  ( 109.0695705685734254, 106.4195705685780524, 7.000000000000249578 ) ) ;
#14340=ORIENTED_EDGE ( 'NONE', *, *, #23394, .F. ) ;
#14343=ORIENTED_EDGE ( 'NONE', *, *, #35908, .T. ) ;
#14379=CARTESIAN_POINT ( 'NONE',  ( 1.798435537469519230E-14, -1.196353617197826191E-13, -44.99999999999999289 ) ) ;
#14383=CARTESIAN_POINT ( 'NONE',  ( 106.4195705685756792, -106.4195705685758213, 9.999999999999671374 ) ) ;
#14389=EDGE_LOOP ( 'NONE', ( #28326, #7818, #10347, #5693 ) ) ;
#14414=LINE ( 'NONE', #37077, #23071 ) ;
#14536=LINE ( 'NONE', #955, #41600 ) ;
#14551=PLANE ( 'NONE',  #2537 ) ;
#14597=DIRECTION ( 'NONE',  ( 0.000000000000000000, 0.000000000000000000, 1.000000000000000000 ) ) ;
#14832=CARTESIAN_POINT ( 'NONE',  ( -3.996523416598931009E-15, 2.658563593772952281E-14, 10.00000000000000178 ) ) ;
#14845=DIRECTION ( 'NONE',  ( 1.000000000000000000, 0.000000000000000000, -6.546126324440850663E-16 ) ) ;
#14850=DIRECTION ( 'NONE',  ( -3.996523416598930318E-16, 2.658563593772947863E-15, 1.000000000000000000 ) ) ;
#14862=AXIS2_PLACEMENT_3D ( 'NONE', #18128, #21617, #30951 ) ;
#14883=SHAPE_DEFINITION_REPRESENTATION ( #13411, #9026 ) ;
#14955=PLANE ( 'NONE',  #42083 ) ;
#15077=AXIS2_PLACEMENT_3D ( 'NONE', #38459, #34775, #42151 ) ;
#15103=CIRCLE ( 'NONE', #26909, 19.99999999999989342 ) ;
#15129=EDGE_CURVE ( 'NONE', #17775, #15772, #6122, .T. ) ;
#15179=FACE_BOUND ( 'NONE', #15973, .T. ) ;
#15265=ORIENTED_EDGE ( 'NONE', *, *, #24391, .T. ) ;
#15266=DIRECTION ( 'NONE',  ( 1.000000000000000000, -1.373900992973642263E-15, 0.000000000000000000 ) ) ;
#15278=CIRCLE ( 'NONE', #28501, 129.9999999999993463 ) ;
#15332=EDGE_CURVE ( 'NONE', #7188, #24964, #13858, .T. ) ;
#15390=EDGE_CURVE ( 'NONE', #239, #24680, #15278, .T. ) ;
#15412=ORIENTED_EDGE ( 'NONE', *, *, #2004, .F. ) ;
#15437=ORIENTED_EDGE ( 'NONE', *, *, #9828, .F. ) ;
#15506=ORIENTED_EDGE ( 'NONE', *, *, #5147, .F. ) ;
#15568=DIRECTION ( 'NONE',  ( 1.000000000000000000, -1.373900992973642263E-15, -4.525365589504737954E-16 ) ) ;
#15573=( NAMED_UNIT ( * ) SI_UNIT ( $, .STERADIAN. ) SOLID_ANGLE_UNIT ( ) );
#15593=DIRECTION ( 'NONE',  ( -3.996523416598930318E-16, 2.658563593772947863E-15, 1.000000000000000000 ) ) ;
#15594=CARTESIAN_POINT ( 'NONE',  ( 1.039096088315723056E-14, -6.912265343809663812E-14, -26.00000000000000355 ) ) ;
#15659=LINE ( 'NONE', #42873, #16956 ) ;
#15671=CARTESIAN_POINT ( 'NONE',  ( -147.8499999999987438, -2.957510437470159335E-13, 10.00000000000004441 ) ) ;
#15683=ORIENTED_EDGE ( 'NONE', *, *, #15390, .F. ) ;
#15695=FACE_OUTER_BOUND ( 'NONE', #33786, .T. ) ;
#15708=CARTESIAN_POINT ( 'NONE',  ( 19.99999999999990408, -9.415137969927464789E-14, -26.00000000000001066 ) ) ;
#15769=CIRCLE ( 'NONE', #33149, 130.0000000000013927 ) ;
#15772=VERTEX_POINT ( 'NONE', #7243 ) ;
#15809=DIRECTION ( 'NONE',  ( 7.831767060816205381E-16, -2.691216939431690932E-15, 1.000000000000000000 ) ) ;
#15835=CARTESIAN_POINT ( 'NONE',  ( -12.49999999999991829, -1.009307908086780017E-13, -44.99999999999998579 ) ) ;
#15879=CARTESIAN_POINT ( 'NONE',  ( 102.9999999999993321, -2.372200916521104037E-13, -32.00000000000000000 ) ) ;
#15973=EDGE_LOOP ( 'NONE', ( #4254, #26899 ) ) ;
#15982=ORIENTED_EDGE ( 'NONE', *, *, #31090, .F. ) ;
#15988=VECTOR ( 'NONE', #24144, 1000.000000000000000 ) ;
#16012=AXIS2_PLACEMENT_3D ( 'NONE', #1258, #34205, #27909 ) ;
#16045=AXIS2_PLACEMENT_3D ( 'NONE', #18895, #25421, #42586 ) ;
#16182=ORIENTED_EDGE ( 'NONE', *, *, #24949, .F. ) ;
#16200=CARTESIAN_POINT ( 'NONE',  ( -12.49999999999998401, -9.428438182424557364E-14, -40.00000000000000711 ) ) ;
#16243=ORIENTED_EDGE ( 'NONE', *, *, #8607, .T. ) ;
#16254=VERTEX_POINT ( 'NONE', #11356 ) ;
#16312=CIRCLE ( 'NONE', #3733, 2.649999999999971934 ) ;
#16314=DIRECTION ( 'NONE',  ( -3.996523416598930318E-16, 2.658563593772947863E-15, 1.000000000000000000 ) ) ;
#16342=ORIENTED_EDGE ( 'NONE', *, *, #18809, .F. ) ;
#16467=ORIENTED_EDGE ( 'NONE', *, *, #2465, .F. ) ;
#16480=LINE ( 'NONE', #15835, #8768 ) ;
#16510=FACE_OUTER_BOUND ( 'NONE', #37940, .T. ) ;
#16511=ORIENTED_EDGE ( 'NONE', *, *, #39033, .T. ) ;
#16517=ORIENTED_EDGE ( 'NONE', *, *, #18377, .F. ) ;
#16524=CARTESIAN_POINT ( 'NONE',  ( 109.0695705685734254, 106.4195705685780524, 10.00000000000025224 ) ) ;
#16560=ADVANCED_FACE ( 'NONE', ( #21985 ), #5782, .F. ) ;
#16616=ORIENTED_EDGE ( 'NONE', *, *, #30450, .T. ) ;
#16632=DIRECTION ( 'NONE',  ( 3.996523416598930318E-16, -2.658563593772947863E-15, -1.000000000000000000 ) ) ;
#16642=ORIENTED_EDGE ( 'NONE', *, *, #15332, .T. ) ;
#16650=ORIENTED_EDGE ( 'NONE', *, *, #25649, .T. ) ;
#16801=ORIENTED_EDGE ( 'NONE', *, *, #12311, .F. ) ;
#16813=AXIS2_PLACEMENT_3D ( 'NONE', #13082, #26379, #39645 ) ;
#16827=CARTESIAN_POINT ( 'NONE',  ( -103.7695705685742240, -106.4195705685773135, 9.999999999999749534 ) ) ;
#16837=CARTESIAN_POINT ( 'NONE',  ( 2.027755760259328333E-13, -150.5000000000013642, 9.999999999999587885 ) ) ;
#16848=ORIENTED_EDGE ( 'NONE', *, *, #130, .T. ) ;
#16904=DIRECTION ( 'NONE',  ( 1.000000000000000000, 0.000000000000000000, -6.546126324440832913E-16 ) ) ;
#16956=VECTOR ( 'NONE', #6445, 1000.000000000000000 ) ;
#17010=CIRCLE ( 'NONE', #25364, 2.649999999999979039 ) ;
#17031=CIRCLE ( 'NONE', #41365, 2.649999999999971934 ) ;
#17087=ORIENTED_EDGE ( 'NONE', *, *, #39864, .F. ) ;
#17114=CARTESIAN_POINT ( 'NONE',  ( 150.4999999999986926, 1.396217360982896810E-12, 9.999999999999962697 ) ) ;
#17117=PLANE ( 'NONE',  #21626 ) ;
#17126=AXIS2_PLACEMENT_3D ( 'NONE', #11610, #42478, #12623 ) ;
#17144=ORIENTED_EDGE ( 'NONE', *, *, #38290, .F. ) ;
#17167=FACE_OUTER_BOUND ( 'NONE', #28740, .T. ) ;
#17196=DIRECTION ( 'NONE',  ( 1.000000000000000000, -1.373900992973641868E-15, -6.546126324440886161E-16 ) ) ;
#17215=ORIENTED_EDGE ( 'NONE', *, *, #29944, .T. ) ;
#17304=CARTESIAN_POINT ( 'NONE',  ( 106.4195705685756792, -106.4195705685758213, 9.999999999999669598 ) ) ;
#17340=AXIS2_PLACEMENT_3D ( 'NONE', #18070, #28069, #5125 ) ;
#17351=ORIENTED_EDGE ( 'NONE', *, *, #31600, .F. ) ;
#17360=CARTESIAN_POINT ( 'NONE',  ( 139.4999999999992610, -1.479897297339870344E-13, 9.999999999999946709 ) ) ;
#17382=ORIENTED_EDGE ( 'NONE', *, *, #19309, .F. ) ;
#17407=PRODUCT_DEFINITION_CONTEXT ( 'detailed design', #32827, 'design' ) ;
#17414=CARTESIAN_POINT ( 'NONE',  ( -150.4999999999986926, -2.921102061156358310E-13, 10.00000000000004619 ) ) ;
#17451=DIRECTION ( 'NONE',  ( 3.996523416598930318E-16, -2.658563593772947863E-15, -1.000000000000000000 ) ) ;
#17503=CARTESIAN_POINT ( 'NONE',  ( 102.9999999999993321, -2.372200916521103027E-13, -40.00000000000000000 ) ) ;
#17538=DIRECTION ( 'NONE',  ( -3.996523416598930318E-16, 2.658563593772947863E-15, 1.000000000000000000 ) ) ;
#17555=DIRECTION ( 'NONE',  ( 1.000000000000000000, -1.373900992973641868E-15, -6.546126324440886161E-16 ) ) ;
#17559=ORIENTED_EDGE ( 'NONE', *, *, #39033, .F. ) ;
#17574=VERTEX_POINT ( 'NONE', #20871 ) ;
#17582=ORIENTED_EDGE ( 'NONE', *, *, #35139, .F. ) ;
#17593=LINE ( 'NONE', #38259, #1669 ) ;
#17605=ORIENTED_EDGE ( 'NONE', *, *, #21702, .T. ) ;
#17653=AXIS2_PLACEMENT_3D ( 'NONE', #39012, #32265, #35730 ) ;
#17671=ORIENTED_EDGE ( 'NONE', *, *, #19082, .F. ) ;
#17695=LINE ( 'NONE', #20532, #4724 ) ;
#17701=DIRECTION ( 'NONE',  ( -3.996523416598930318E-16, 2.658563593772947863E-15, 1.000000000000000000 ) ) ;
#17775=VERTEX_POINT ( 'NONE', #31722 ) ;
#17820=CARTESIAN_POINT ( 'NONE',  ( 2.164352920501969098E-14, -1.058809993658036520E-13, -40.00000000000000000 ) ) ;
#17828=LINE ( 'NONE', #21551, #23741 ) ;
#17835=UNCERTAINTY_MEASURE_WITH_UNIT (LENGTH_MEASURE( 1.000000000000000082E-05 ), #25202, 'distance_accuracy_value', 'NONE');
#17862=AXIS2_PLACEMENT_3D ( 'NONE', #35417, #5942, #25418 ) ;
#17865=DIRECTION ( 'NONE',  ( 1.000000000000000000, -1.373900992973641671E-15, -3.895519384649692070E-16 ) ) ;
#17892=( GEOMETRIC_REPRESENTATION_CONTEXT ( 3 ) GLOBAL_UNCERTAINTY_ASSIGNED_CONTEXT ( ( #42660 ) ) GLOBAL_UNIT_ASSIGNED_CONTEXT ( ( #42139, #8786, #22145 ) ) REPRESENTATION_CONTEXT ( 'NONE', 'WORKASPACE' ) );
#17894=CIRCLE ( 'NONE', #3170, 2.649999999999971934 ) ;
#17904=CARTESIAN_POINT ( 'NONE',  ( -12.49999999999998401, -9.428438182424551053E-14, -45.00000000000000000 ) ) ;
#17911=FACE_BOUND ( 'NONE', #42096, .T. ) ;
#17936=DIRECTION ( 'NONE',  ( -3.996523416598930318E-16, 2.658563593772947863E-15, 1.000000000000000000 ) ) ;
#17956=AXIS2_PLACEMENT_3D ( 'NONE', #17820, #37187, #7741 ) ;
#18032=AXIS2_PLACEMENT_3D ( 'NONE', #26208, #35768, #32309 ) ;
#18038=ORIENTED_EDGE ( 'NONE', *, *, #33064, .T. ) ;
#18070=CARTESIAN_POINT ( 'NONE',  ( 2.039745330509125010E-13, -150.5000000000013642, 6.999999999999586109 ) ) ;
#18076=LINE ( 'NONE', #38081, #30196 ) ;
#18077=DIRECTION ( 'NONE',  ( -3.996523416598930318E-16, 2.658563593772947863E-15, 1.000000000000000000 ) ) ;
#18098=VERTEX_POINT ( 'NONE', #21471 ) ;
#18114=DIRECTION ( 'NONE',  ( 1.000000000000000000, -1.373900992973641671E-15, -3.895519384649692070E-16 ) ) ;
#18116=ORIENTED_EDGE ( 'NONE', *, *, #21265, .F. ) ;
#18127=ORIENTED_EDGE ( 'NONE', *, *, #35189, .F. ) ;
#18128=CARTESIAN_POINT ( 'NONE',  ( -150.4999999999986926, -3.000858968969551636E-13, 7.000000000000042633 ) ) ;
#18193=DIRECTION ( 'NONE',  ( -3.996523416598930318E-16, 2.658563593772947863E-15, 1.000000000000000000 ) ) ;
#18278=FACE_OUTER_BOUND ( 'NONE', #35887, .T. ) ;
#18326=AXIS2_PLACEMENT_3D ( 'NONE', #29499, #25820, #26232 ) ;
#18360=DIRECTION ( 'NONE',  ( -1.000000000000000000, 1.373900992973642066E-15, 3.979293995072266947E-16 ) ) ;
#18377=EDGE_CURVE ( 'NONE', #11054, #15772, #26417, .T. ) ;
#18406=EDGE_CURVE ( 'NONE', #2151, #21317, #39554, .T. ) ;
#18415=ORIENTED_EDGE ( 'NONE', *, *, #15332, .F. ) ;
#18440=( LENGTH_UNIT ( ) NAMED_UNIT ( * ) SI_UNIT ( .MILLI., .METRE. ) );
#18458=FACE_BOUND ( 'NONE', #32525, .T. ) ;
#18471=CARTESIAN_POINT ( 'NONE',  ( -106.4195705685741871, -106.4195705685773135, 9.999999999999753086 ) ) ;
#18498=ORIENTED_EDGE ( 'NONE', *, *, #18569, .F. ) ;
#18548=CIRCLE ( 'NONE', #17126, 139.4999999999992610 ) ;
#18569=EDGE_CURVE ( 'NONE', #4344, #38954, #17695, .T. ) ;
#18603=DIRECTION ( 'NONE',  ( 3.996523416598930318E-16, -2.658563593772947863E-15, -1.000000000000000000 ) ) ;
#18656=ADVANCED_FACE ( 'NONE', ( #8921 ), #38790, .F. ) ;
#18670=EDGE_LOOP ( 'NONE', ( #30660, #2270, #28261, #5740 ) ) ;
#18671=( NAMED_UNIT ( * ) PLANE_ANGLE_UNIT ( ) SI_UNIT ( $, .RADIAN. ) );
#18703=FACE_OUTER_BOUND ( 'NONE', #23639, .T. ) ;
#18764=CARTESIAN_POINT ( 'NONE',  ( 1.039096088315723056E-14, -6.912265343809663812E-14, -26.00000000000000355 ) ) ;
#18809=EDGE_CURVE ( 'NONE', #20992, #25091, #28582, .T. ) ;
#18849=AXIS2_PLACEMENT_3D ( 'NONE', #41917, #25384, #12698 ) ;
#18872=SURFACE_SIDE_STYLE ('',( #11873 ) ) ;
#18895=CARTESIAN_POINT ( 'NONE',  ( -3.996523416598931009E-15, 2.658563593772952281E-14, 10.00000000000000178 ) ) ;
#18900=DIRECTION ( 'NONE',  ( 1.000000000000000000, 0.000000000000000000, -6.546126324440850663E-16 ) ) ;
#18908=CARTESIAN_POINT ( 'NONE',  ( 1.039096088315723056E-14, -6.912265343809663812E-14, -26.00000000000000355 ) ) ;
#18924=CARTESIAN_POINT ( 'NONE',  ( 2.039745330509125010E-13, -150.5000000000013642, 6.999999999999586109 ) ) ;
#18933=AXIS2_PLACEMENT_3D ( 'NONE', #18924, #22196, #32390 ) ;
#18976=ORIENTED_EDGE ( 'NONE', *, *, #33861, .F. ) ;
#18995=CIRCLE ( 'NONE', #38456, 2.649999999999971934 ) ;
#19047=VERTEX_POINT ( 'NONE', #11240 ) ;
#19061=CARTESIAN_POINT ( 'NONE',  ( 109.0695705685756565, -106.4195705685758213, 6.999999999999666933 ) ) ;
#19082=EDGE_CURVE ( 'NONE', #41484, #40947, #8284, .T. ) ;
#19121=CARTESIAN_POINT ( 'NONE',  ( 1.039096088315723056E-14, -6.912265343809663812E-14, -26.00000000000000355 ) ) ;
#19128=DIRECTION ( 'NONE',  ( -3.996523416598930318E-16, 2.658563593772947863E-15, 1.000000000000000000 ) ) ;
#19156=CARTESIAN_POINT ( 'NONE',  ( 106.4195705685756792, -106.4195705685758213, 9.999999999999669598 ) ) ;
#19309=EDGE_CURVE ( 'NONE', #32279, #11569, #38914, .T. ) ;
#19310=FACE_OUTER_BOUND ( 'NONE', #11352, .T. ) ;
#19340=CIRCLE ( 'NONE', #1888, 2.649999999999957723 ) ;
#19368=VERTEX_POINT ( 'NONE', #13606 ) ;
#19401=CIRCLE ( 'NONE', #21506, 1.999999999999988010 ) ;
#19408=CARTESIAN_POINT ( 'NONE',  ( 2.650000000000176215, -150.5000000000013642, 9.999999999999586109 ) ) ;
#19412=CYLINDRICAL_SURFACE ( 'NONE', #35017, 2.649999999999971934 ) ;
#19426=DIRECTION ( 'NONE',  ( 1.000000000000000000, -1.373900992973641868E-15, -6.546126324440886161E-16 ) ) ;
#19432=ORIENTED_EDGE ( 'NONE', *, *, #25527, .F. ) ;
#19465=DIRECTION ( 'NONE',  ( -3.996523416598930318E-16, 2.658563593772947863E-15, 1.000000000000000000 ) ) ;
#19509=FACE_OUTER_BOUND ( 'NONE', #28644, .T. ) ;
#19518=CARTESIAN_POINT ( 'NONE',  ( 2.164352920501969098E-14, -1.058809993658036520E-13, -40.00000000000000000 ) ) ;
#19671=CARTESIAN_POINT ( 'NONE',  ( -19.99999999999988276, -4.164463357862395064E-14, -25.99999999999999645 ) ) ;
#19696=EDGE_LOOP ( 'NONE', ( #1612, #37638 ) ) ;
#19699=CARTESIAN_POINT ( 'NONE',  ( -153.1499999999986699, -2.921326824731410475E-13, 10.00000000000004441 ) ) ;
#19713=ORIENTED_EDGE ( 'NONE', *, *, #36497, .F. ) ;
#19780=CARTESIAN_POINT ( 'NONE',  ( -109.0695705685749175, 106.4195705685765745, 10.00000000000033751 ) ) ;
#19855=ORIENTED_EDGE ( 'NONE', *, *, #31707, .T. ) ;
#19867=ADVANCED_FACE ( 'NONE', ( #6331 ), #27073, .F. ) ;
#19868=ORIENTED_EDGE ( 'NONE', *, *, #29944, .F. ) ;
#19900=CARTESIAN_POINT ( 'NONE',  ( 23.00000000000001421, -1.165156337948619932E-13, -39.99999999999999289 ) ) ;
#19948=ORIENTED_EDGE ( 'NONE', *, *, #31707, .F. ) ;
#19995=CIRCLE ( 'NONE', #1130, 12.49999999999993427 ) ;
#20013=EDGE_CURVE ( 'NONE', #42401, #32464, #561, .T. ) ;
#20048=ORIENTED_EDGE ( 'NONE', *, *, #11236, .T. ) ;
#20079=AXIS2_PLACEMENT_3D ( 'NONE', #14379, #7809, #27249 ) ;
#20142=EDGE_CURVE ( 'NONE', #32971, #17775, #9132, .T. ) ;
#20157=DIRECTION ( 'NONE',  ( 1.000000000000000000, -1.373900992973641868E-15, -6.546126324440886161E-16 ) ) ;
#20180=EDGE_LOOP ( 'NONE', ( #24785, #19855, #29231, #12919 ) ) ;
#20238=DIRECTION ( 'NONE',  ( -3.996523416598930318E-16, 2.658563593772947863E-15, 1.000000000000000000 ) ) ;
#20249=VERTEX_POINT ( 'NONE', #2977 ) ;
#20297=CYLINDRICAL_SURFACE ( 'NONE', #6721, 22.99999999999987921 ) ;
#20298=CIRCLE ( 'NONE', #10510, 139.4999999999992610 ) ;
#20300=CIRCLE ( 'NONE', #32100, 2.649999999999971934 ) ;
#20331=CARTESIAN_POINT ( 'NONE',  ( 1.039096088315723056E-14, -6.912265343809663812E-14, -26.00000000000000355 ) ) ;
#20355=ADVANCED_FACE ( 'NONE', ( #36817 ), #9776, .F. ) ;
#20393=DIRECTION ( 'NONE',  ( 3.996523416598993920E-16, 2.658563593772947074E-15, 1.000000000000000000 ) ) ;
#20437=DIRECTION ( 'NONE',  ( 3.996523416598930318E-16, -2.658563593772947863E-15, -1.000000000000000000 ) ) ;
#20458=ORIENTED_EDGE ( 'NONE', *, *, #37223, .F. ) ;
#20506=DIRECTION ( 'NONE',  ( -3.996523416598930318E-16, 2.658563593772947863E-15, 1.000000000000000000 ) ) ;
#20532=CARTESIAN_POINT ( 'NONE',  ( -125.9999999999995026, 1.156432136281054424E-12, 369.6955262170048400 ) ) ;
#20545=CARTESIAN_POINT ( 'NONE',  ( 103.7695705685734708, 106.4195705685780382, 10.00000000000025224 ) ) ;
#20551=VECTOR ( 'NONE', #22443, 1000.000000000000000 ) ;
#20598=ADVANCED_FACE ( 'NONE', ( #25709 ), #25279, .F. ) ;
#20604=AXIS2_PLACEMENT_3D ( 'NONE', #22997, #22561, #26024 ) ;
#20652=STYLED_ITEM ( 'NONE', ( #28872 ), #13589 ) ;
#20662=DIRECTION ( 'NONE',  ( 3.996523416598930318E-16, -2.658563593772947863E-15, -1.000000000000000000 ) ) ;
#20683=VERTEX_POINT ( 'NONE', #21804 ) ;
#20718=AXIS2_PLACEMENT_3D ( 'NONE', #5480, #18193, #31889 ) ;
#20740=EDGE_LOOP ( 'NONE', ( #17087, #37472, #28239, #13603 ) ) ;
#20746=FACE_BOUND ( 'NONE', #39737, .T. ) ;
#20826=EDGE_LOOP ( 'NONE', ( #9565, #31175, #35307, #24152 ) ) ;
#20871=CARTESIAN_POINT ( 'NONE',  ( 153.1499999999986414, 1.392576523351516607E-12, 9.999999999999960920 ) ) ;
#20872=AXIS2_PLACEMENT_3D ( 'NONE', #28503, #2045, #34574 ) ;
#20880=CARTESIAN_POINT ( 'NONE',  ( -2.841217984690893843E-16, 1.478917074864463474E-14, 1.999999999999980904 ) ) ;
#20926=VERTEX_POINT ( 'NONE', #14308 ) ;
#20992=VERTEX_POINT ( 'NONE', #43006 ) ;
#20997=EDGE_LOOP ( 'NONE', ( #9604, #5623, #39024, #9219 ) ) ;
#21011=ORIENTED_EDGE ( 'NONE', *, *, #36497, .T. ) ;
#21070=LINE ( 'NONE', #25196, #3970 ) ;
#21084=EDGE_LOOP ( 'NONE', ( #19948, #17382, #16650, #18038 ) ) ;
#21103=ORIENTED_EDGE ( 'NONE', *, *, #12659, .F. ) ;
#21104=CARTESIAN_POINT ( 'NONE',  ( -158.4999999999992042, 2.557839043092172690E-13, 7.000000000000065725 ) ) ;
#21158=DIRECTION ( 'NONE',  ( -1.000000000000000000, 1.373900992973641868E-15, 4.405646923115722869E-16 ) ) ;
#21232=ORIENTED_EDGE ( 'NONE', *, *, #33858, .T. ) ;
#21234=FACE_OUTER_BOUND ( 'NONE', #20740, .T. ) ;
#21241=CIRCLE ( 'NONE', #42772, 2.649999999999971934 ) ;
#21246=EDGE_CURVE ( 'NONE', #12177, #3549, #37291, .T. ) ;
#21262=ORIENTED_EDGE ( 'NONE', *, *, #26144, .T. ) ;
#21265=EDGE_CURVE ( 'NONE', #3549, #12177, #18548, .T. ) ;
#21271=DIRECTION ( 'NONE',  ( -3.996523416598930318E-16, 2.658563593772947863E-15, 1.000000000000000000 ) ) ;
#21317=VERTEX_POINT ( 'NONE', #19408 ) ;
#21387=CYLINDRICAL_SURFACE ( 'NONE', #12672, 2.649999999999971934 ) ;
#21401=DIRECTION ( 'NONE',  ( -3.996523416598930318E-16, 2.658563593772947863E-15, 1.000000000000000000 ) ) ;
#21458=PRODUCT_CONTEXT ( 'NONE', #40067, 'mechanical' ) ;
#21471=CARTESIAN_POINT ( 'NONE',  ( 106.9999999999993321, -2.424707662641754077E-13, -32.00000000000000000 ) ) ;
#21488=LINE ( 'NONE', #13835, #35252 ) ;
#21499=ORIENTED_EDGE ( 'NONE', *, *, #12439, .F. ) ;
#21506=AXIS2_PLACEMENT_3D ( 'NONE', #22376, #25650, #2665 ) ;
#21551=CARTESIAN_POINT ( 'NONE',  ( -153.1499999999986414, -2.881448370824816841E-13, 10.00000000000004619 ) ) ;
#21568=DIRECTION ( 'NONE',  ( -3.996523416598930318E-16, 2.658563593772947863E-15, 1.000000000000000000 ) ) ;
#21596=ORIENTED_EDGE ( 'NONE', *, *, #30551, .T. ) ;
#21605=DIRECTION ( 'NONE',  ( -3.996523416598930318E-16, 2.658563593772947863E-15, 1.000000000000000000 ) ) ;
#21617=DIRECTION ( 'NONE',  ( -3.996523416598930318E-16, 2.658563593772947863E-15, 1.000000000000000000 ) ) ;
#21626=AXIS2_PLACEMENT_3D ( 'NONE', #40189, #20393, #33653 ) ;
#21654=CIRCLE ( 'NONE', #18849, 125.9999999999993605 ) ;
#21702=EDGE_CURVE ( 'NONE', #22603, #27398, #17010, .T. ) ;
#21720=SHAPE_REPRESENTATION_RELATIONSHIP ( 'NONE' , 'NONE' ,  #9026, #4160 ) ;
#21723=ORIENTED_EDGE ( 'NONE', *, *, #26998, .T. ) ;
#21804=CARTESIAN_POINT ( 'NONE',  ( -147.8499999999987438, -3.037267345283352157E-13, 7.000000000000041744 ) ) ;
#21891=EDGE_CURVE ( 'NONE', #25432, #14258, #35128, .T. ) ;
#21919=DIRECTION ( 'NONE',  ( 3.996523416598930318E-16, -2.658563593772947863E-15, -1.000000000000000000 ) ) ;
#21934=ORIENTED_EDGE ( 'NONE', *, *, #11645, .T. ) ;
#21941=FACE_BOUND ( 'NONE', #33829, .T. ) ;
#21952=VERTEX_POINT ( 'NONE', #31416 ) ;
#21977=CARTESIAN_POINT ( 'NONE',  ( 1.039096088315723056E-14, -6.912265343809663812E-14, -26.00000000000000355 ) ) ;
#21985=FACE_OUTER_BOUND ( 'NONE', #22609, .T. ) ;
#21998=DIRECTION ( 'NONE',  ( -3.996523416598930318E-16, 2.658563593772947863E-15, 1.000000000000000000 ) ) ;
#22110=ORIENTED_EDGE ( 'NONE', *, *, #37465, .F. ) ;
#22114=EDGE_CURVE ( 'NONE', #16254, #20926, #16312, .T. ) ;
#22116=DIRECTION ( 'NONE',  ( -3.996523416598930318E-16, 2.658563593772947863E-15, 1.000000000000000000 ) ) ;
#22120=AXIS2_PLACEMENT_3D ( 'NONE', #22194, #35447, #35227 ) ;
#22145=( NAMED_UNIT ( * ) SI_UNIT ( $, .STERADIAN. ) SOLID_ANGLE_UNIT ( ) );
#22194=CARTESIAN_POINT ( 'NONE',  ( 2.027755760259328333E-13, -150.5000000000013642, 9.999999999999587885 ) ) ;
#22196=DIRECTION ( 'NONE',  ( -3.996523416598930318E-16, 2.658563593772947863E-15, 1.000000000000000000 ) ) ;
#22271=VECTOR ( 'NONE', #29334, 1000.000000000000000 ) ;
#22293=FACE_OUTER_BOUND ( 'NONE', #11884, .T. ) ;
#22327=CARTESIAN_POINT ( 'NONE',  ( -158.5000000000000284, 2.597717496998778441E-13, 6.999999999999939604 ) ) ;
#22347=ORIENTED_EDGE ( 'NONE', *, *, #23450, .T. ) ;
#22376=CARTESIAN_POINT ( 'NONE',  ( 104.9999999999993321, -2.293336392629658115E-13, -32.00000000000000000 ) ) ;
#22396=CARTESIAN_POINT ( 'NONE',  ( -150.4999999999986926, -2.921102061156358310E-13, 10.00000000000004619 ) ) ;
#22405=CARTESIAN_POINT ( 'NONE',  ( -2.107686228591307694E-13, 150.5000000000013642, 10.00000000000041744 ) ) ;
#22443=DIRECTION ( 'NONE',  ( 3.996523416598930318E-16, -2.658563593772947863E-15, -1.000000000000000000 ) ) ;
#22444=AXIS2_PLACEMENT_3D ( 'NONE', #33451, #3539, #38437 ) ;
#22476=DIRECTION ( 'NONE',  ( 3.996523416598930318E-16, -2.658563593772947863E-15, -1.000000000000000000 ) ) ;
#22507=ORIENTED_EDGE ( 'NONE', *, *, #40139, .T. ) ;
#22561=DIRECTION ( 'NONE',  ( -3.996523416598930318E-16, 2.658563593772947863E-15, 1.000000000000000000 ) ) ;
#22568=ORIENTED_EDGE ( 'NONE', *, *, #2638, .F. ) ;
#22582=CARTESIAN_POINT ( 'NONE',  ( 106.4195705685756792, -106.4195705685758213, 6.999999999999667821 ) ) ;
#22595=DIRECTION ( 'NONE',  ( 3.996523416598930318E-16, -2.658563593772947863E-15, -1.000000000000000000 ) ) ;
#22603=VERTEX_POINT ( 'NONE', #9076 ) ;
#22609=EDGE_LOOP ( 'NONE', ( #38916, #21232, #25168, #37530 ) ) ;
#22664=ORIENTED_EDGE ( 'NONE', *, *, #401, .F. ) ;
#22746=EDGE_LOOP ( 'NONE', ( #39217, #32736, #41243, #27231 ) ) ;
#22786=VERTEX_POINT ( 'NONE', #40235 ) ;
#22794=CARTESIAN_POINT ( 'NONE',  ( 106.4195705685734623, 106.4195705685780524, 10.00000000000025224 ) ) ;
#22798=DIRECTION ( 'NONE',  ( -3.996523416598930318E-16, 2.658563593772947863E-15, 1.000000000000000000 ) ) ;
#22801=CARTESIAN_POINT ( 'NONE',  ( 106.4195705685734623, 106.4195705685780524, 10.00000000000025224 ) ) ;
#22966=DIRECTION ( 'NONE',  ( -3.996523416598930318E-16, 2.658563593772947863E-15, 1.000000000000000000 ) ) ;
#22997=CARTESIAN_POINT ( 'NONE',  ( 150.4999999999986926, 1.396217360982896810E-12, 9.999999999999960920 ) ) ;
#23008=CIRCLE ( 'NONE', #13211, 2.649999999999957723 ) ;
#23016=DIRECTION ( 'NONE',  ( -3.996523416598930318E-16, 2.658563593772947863E-15, 1.000000000000000000 ) ) ;
#23022=ORIENTED_EDGE ( 'NONE', *, *, #10929, .T. ) ;
#23071=VECTOR ( 'NONE', #26842, 1000.000000000000000 ) ;
#23186=ORIENTED_EDGE ( 'NONE', *, *, #8514, .F. ) ;
#23268=CARTESIAN_POINT ( 'NONE',  ( -2.797566391619251075E-15, 1.860994515641065082E-14, 7.000000000000002665 ) ) ;
#23286=AXIS2_PLACEMENT_3D ( 'NONE', #17114, #30403, #17555 ) ;
#23334=ORIENTED_EDGE ( 'NONE', *, *, #20142, .T. ) ;
#23353=VECTOR ( 'NONE', #24246, 1000.000000000000000 ) ;
#23367=DIRECTION ( 'NONE',  ( 1.000000000000000000, 0.000000000000000000, -6.546126324440847704E-16 ) ) ;
#23394=EDGE_CURVE ( 'NONE', #32776, #4344, #5304, .T. ) ;
#23450=EDGE_CURVE ( 'NONE', #32776, #20249, #21488, .T. ) ;
#23455=EDGE_LOOP ( 'NONE', ( #18415, #10596, #22507, #9681 ) ) ;
#23479=VERTEX_POINT ( 'NONE', #42929 ) ;
#23494=ORIENTED_EDGE ( 'NONE', *, *, #401, .T. ) ;
#23585=FACE_OUTER_BOUND ( 'NONE', #4181, .T. ) ;
#23611=CIRCLE ( 'NONE', #17956, 129.9999999999993463 ) ;
#23630=VECTOR ( 'NONE', #41861, 1000.000000000000000 ) ;
#23639=EDGE_LOOP ( 'NONE', ( #16801, #8329, #30742, #35970 ) ) ;
#23640=CARTESIAN_POINT ( 'NONE',  ( 106.4195705685756792, -106.4195705685758213, 6.999999999999667821 ) ) ;
#23650=PRODUCT_DEFINITION ( 'UNKNOWN', '', #12151, #17407 ) ;
#23657=ORIENTED_EDGE ( 'NONE', *, *, #12439, .T. ) ;
#23677=ORIENTED_EDGE ( 'NONE', *, *, #36760, .F. ) ;
#23741=VECTOR ( 'NONE', #28061, 1000.000000000000000 ) ;
#23793=DIRECTION ( 'NONE',  ( 1.000000000000000000, -1.373900992973642263E-15, -3.996523416598957436E-16 ) ) ;
#23794=LINE ( 'NONE', #16827, #37236 ) ;
#23873=ORIENTED_EDGE ( 'NONE', *, *, #29230, .T. ) ;
#23874=DIRECTION ( 'NONE',  ( -3.996523416598930318E-16, 2.658563593772947863E-15, 1.000000000000000000 ) ) ;
#23877=DIRECTION ( 'NONE',  ( 1.000000000000000000, -1.373900992973641868E-15, -3.273063162220443081E-16 ) ) ;
#23893=VERTEX_POINT ( 'NONE', #41153 ) ;
#23923=LINE ( 'NONE', #10148, #15988 ) ;
#23944=VERTEX_POINT ( 'NONE', #15879 ) ;
#23950=CARTESIAN_POINT ( 'NONE',  ( -2.650000000000202860, 150.5000000000013642, 7.000000000000418332 ) ) ;
#23976=AXIS2_PLACEMENT_3D ( 'NONE', #33443, #23874, #16904 ) ;
#24085=CARTESIAN_POINT ( 'NONE',  ( 4.858130855304160865E-15, 5.778671572660278980E-15, 2.000000000000001776 ) ) ;
#24134=DIRECTION ( 'NONE',  ( -3.996523416598930318E-16, 2.658563593772947863E-15, 1.000000000000000000 ) ) ;
#24140=DIRECTION ( 'NONE',  ( 3.996523416598930318E-16, -2.658563593772947863E-15, -1.000000000000000000 ) ) ;
#24144=DIRECTION ( 'NONE',  ( -3.996523416598930318E-16, 2.658563593772947863E-15, 1.000000000000000000 ) ) ;
#24152=ORIENTED_EDGE ( 'NONE', *, *, #15129, .F. ) ;
#24214=LINE ( 'NONE', #34201, #27506 ) ;
#24231=FACE_BOUND ( 'NONE', #26034, .T. ) ;
#24235=CARTESIAN_POINT ( 'NONE',  ( -106.4195705685749402, 106.4195705685765745, 10.00000000000033573 ) ) ;
#24246=DIRECTION ( 'NONE',  ( -3.996523416598930318E-16, 2.658563593772947863E-15, 1.000000000000000000 ) ) ;
#24257=CARTESIAN_POINT ( 'NONE',  ( 1.598609366639573350E-14, -1.063425437509180407E-13, -40.00000000000000000 ) ) ;
#24291=CYLINDRICAL_SURFACE ( 'NONE', #4449, 2.649999999999957723 ) ;
#24327=AXIS2_PLACEMENT_3D ( 'NONE', #32948, #33389, #3474 ) ;
#24359=DIRECTION ( 'NONE',  ( 3.892440008040322386E-16, -2.658563593772947863E-15, -1.000000000000000000 ) ) ;
#24373=ADVANCED_FACE ( 'NONE', ( #6938 ), #20297, .T. ) ;
#24391=EDGE_CURVE ( 'NONE', #22786, #20683, #25583, .T. ) ;
#24463=CARTESIAN_POINT ( 'NONE',  ( 106.4195705685756792, -106.4195705685758213, 9.999999999999671374 ) ) ;
#24593=AXIS2_PLACEMENT_3D ( 'NONE', #22794, #13384, #29965 ) ;
#24651=EDGE_CURVE ( 'NONE', #9154, #42975, #36311, .T. ) ;
#24661=ADVANCED_FACE ( 'NONE', ( #16510 ), #9919, .T. ) ;
#24680=VERTEX_POINT ( 'NONE', #40594 ) ;
#24688=ORIENTED_EDGE ( 'NONE', *, *, #7875, .T. ) ;
#24703=ORIENTED_EDGE ( 'NONE', *, *, #2791, .T. ) ;
#24725=DIRECTION ( 'NONE',  ( 1.000000000000000000, -1.373900992973641868E-15, -6.546126324440886161E-16 ) ) ;
#24767=EDGE_LOOP ( 'NONE', ( #4332, #699, #38744, #21499 ) ) ;
#24780=FACE_OUTER_BOUND ( 'NONE', #25715, .T. ) ;
#24785=ORIENTED_EDGE ( 'NONE', *, *, #3638, .F. ) ;
#24801=DIRECTION ( 'NONE',  ( -1.000000000000000000, 1.373900992973642263E-15, 0.000000000000000000 ) ) ;
#24817=DIRECTION ( 'NONE',  ( 1.000000000000000000, -1.373900992973642263E-15, -3.996523416598957436E-16 ) ) ;
#24835=VERTEX_POINT ( 'NONE', #19699 ) ;
#24840=CIRCLE ( 'NONE', #5971, 158.4999999999992042 ) ;
#24949=EDGE_CURVE ( 'NONE', #20926, #16254, #13696, .T. ) ;
#24964=VERTEX_POINT ( 'NONE', #33407 ) ;
#25010=ORIENTED_EDGE ( 'NONE', *, *, #18406, .T. ) ;
#25015=FACE_BOUND ( 'NONE', #2847, .T. ) ;
#25023=AXIS2_PLACEMENT_3D ( 'NONE', #24257, #17936, #28153 ) ;
#25052=CARTESIAN_POINT ( 'NONE',  ( 106.4195705685734623, 106.4195705685780524, 10.00000000000025402 ) ) ;
#25091=VERTEX_POINT ( 'NONE', #11591 ) ;
#25111=AXIS2_PLACEMENT_3D ( 'NONE', #18908, #22595, #42812 ) ;
#25168=ORIENTED_EDGE ( 'NONE', *, *, #12659, .T. ) ;
#25196=CARTESIAN_POINT ( 'NONE',  ( -129.9999999999994884, 1.161927740252948949E-12, 369.6955262170048400 ) ) ;
#25202=( LENGTH_UNIT ( ) NAMED_UNIT ( * ) SI_UNIT ( .MILLI., .METRE. ) );
#25205=VERTEX_POINT ( 'NONE', #2365 ) ;
#25214=FACE_BOUND ( 'NONE', #14054, .T. ) ;
#25250=FACE_OUTER_BOUND ( 'NONE', #29980, .T. ) ;
#25279=CYLINDRICAL_SURFACE ( 'NONE', #27131, 2.649999999999971934 ) ;
#25364=AXIS2_PLACEMENT_3D ( 'NONE', #29472, #19465, #32939 ) ;
#25384=DIRECTION ( 'NONE',  ( -3.892440008040322386E-16, 2.658563593772947863E-15, 1.000000000000000000 ) ) ;
#25418=DIRECTION ( 'NONE',  ( 1.000000000000000000, -1.373900992973642066E-15, -3.979293995072266947E-16 ) ) ;
#25421=DIRECTION ( 'NONE',  ( -3.996523416598930318E-16, 2.658563593772947863E-15, 1.000000000000000000 ) ) ;
#25432=VERTEX_POINT ( 'NONE', #26609 ) ;
#25453=CARTESIAN_POINT ( 'NONE',  ( -142.5000000000000284, 1.627194001049074632E-13, 6.999999999999945821 ) ) ;
#25488=DIRECTION ( 'NONE',  ( 1.000000000000000000, 0.000000000000000000, -6.546126324440850663E-16 ) ) ;
#25515=AXIS2_PLACEMENT_3D ( 'NONE', #17414, #37432, #17196 ) ;
#25527=EDGE_CURVE ( 'NONE', #20683, #22786, #34322, .T. ) ;
#25539=FACE_OUTER_BOUND ( 'NONE', #41909, .T. ) ;
#25583=CIRCLE ( 'NONE', #42250, 2.649999999999957723 ) ;
#25588=CARTESIAN_POINT ( 'NONE',  ( 2.164352920501968783E-14, -1.058809993658035131E-13, -39.99999999999997868 ) ) ;
#25597=LINE ( 'NONE', #38635, #1259 ) ;
#25619=FILL_AREA_STYLE_COLOUR ( '', #35946 ) ;
#25641=EDGE_CURVE ( 'NONE', #23944, #31256, #11323, .T. ) ;
#25643=EDGE_LOOP ( 'NONE', ( #29876, #31038, #34307, #22110 ) ) ;
#25647=FACE_BOUND ( 'NONE', #10572, .T. ) ;
#25649=EDGE_CURVE ( 'NONE', #32279, #14258, #1692, .T. ) ;
#25650=DIRECTION ( 'NONE',  ( -3.996523416598930318E-16, 2.658563593772947863E-15, 1.000000000000000000 ) ) ;
#25656=VERTEX_POINT ( 'NONE', #17904 ) ;
#25702=CIRCLE ( 'NONE', #31253, 2.649999999999979039 ) ;
#25709=FACE_OUTER_BOUND ( 'NONE', #21084, .T. ) ;
#25715=EDGE_LOOP ( 'NONE', ( #10471, #14216 ) ) ;
#25773=EDGE_LOOP ( 'NONE', ( #18116, #12065 ) ) ;
#25820=DIRECTION ( 'NONE',  ( -3.996523416598930318E-16, 2.658563593772947863E-15, 1.000000000000000000 ) ) ;
#25889=CIRCLE ( 'NONE', #7039, 1.999999999999988010 ) ;
#25918=CARTESIAN_POINT ( 'NONE',  ( -3.996523416598931009E-15, 2.658563593772952281E-14, 10.00000000000000178 ) ) ;
#26003=ORIENTED_EDGE ( 'NONE', *, *, #11236, .F. ) ;
#26024=DIRECTION ( 'NONE',  ( 1.000000000000000000, -1.373900992973641868E-15, -6.546126324440886161E-16 ) ) ;
#26026=ORIENTED_EDGE ( 'NONE', *, *, #7651, .F. ) ;
#26034=EDGE_LOOP ( 'NONE', ( #17582, #26782 ) ) ;
#26054=VERTEX_POINT ( 'NONE', #37431 ) ;
#26080=FACE_OUTER_BOUND ( 'NONE', #8539, .T. ) ;
#26111=LINE ( 'NONE', #42867, #26981 ) ;
#26144=EDGE_CURVE ( 'NONE', #28359, #17574, #18076, .T. ) ;
#26145=ADVANCED_FACE ( 'NONE', ( #37853 ), #7977, .F. ) ;
#26156=FACE_BOUND ( 'NONE', #33006, .T. ) ;
#26159=DIRECTION ( 'NONE',  ( -3.996523416598930318E-16, 2.658563593772947863E-15, 1.000000000000000000 ) ) ;
#26208=CARTESIAN_POINT ( 'NONE',  ( 104.9999999999993321, -2.293336392629658115E-13, -32.00000000000000000 ) ) ;
#26232=DIRECTION ( 'NONE',  ( 1.000000000000000000, -1.373900992973641868E-15, -3.994789077170585140E-16 ) ) ;
#26251=DIRECTION ( 'NONE',  ( 3.996523416598993920E-16, 2.658563593772947074E-15, 1.000000000000000000 ) ) ;
#26264=DIRECTION ( 'NONE',  ( -1.000000000000000000, 1.373900992973642066E-15, 4.525365589504737954E-16 ) ) ;
#26282=DIRECTION ( 'NONE',  ( -3.996523416598930318E-16, 2.658563593772947863E-15, 1.000000000000000000 ) ) ;
#26307=ADVANCED_FACE ( 'NONE', ( #25250 ), #2692, .F. ) ;
#26316=EDGE_CURVE ( 'NONE', #32971, #11054, #5818, .T. ) ;
#26379=DIRECTION ( 'NONE',  ( 3.996523416598993920E-16, 2.658563593772947074E-15, 1.000000000000000000 ) ) ;
#26417=LINE ( 'NONE', #19671, #36757 ) ;
#26465=DIRECTION ( 'NONE',  ( -3.996523416598930318E-16, 2.658563593772947863E-15, 1.000000000000000000 ) ) ;
#26524=CIRCLE ( 'NONE', #28625, 2.649999999999971934 ) ;
#26602=CARTESIAN_POINT ( 'NONE',  ( -150.4999999999986926, -3.000858968969551636E-13, 7.000000000000042633 ) ) ;
#26609=CARTESIAN_POINT ( 'NONE',  ( 103.7695705685756877, -106.4195705685758213, 9.999999999999669598 ) ) ;
#26614=CARTESIAN_POINT ( 'NONE',  ( -103.7695705685749772, 106.4195705685765745, 7.000000000000336620 ) ) ;
#26628=ORIENTED_EDGE ( 'NONE', *, *, #31090, .T. ) ;
#26782=ORIENTED_EDGE ( 'NONE', *, *, #2791, .F. ) ;
#26813=AXIS2_PLACEMENT_3D ( 'NONE', #6245, #13038, #6033 ) ;
#26842=DIRECTION ( 'NONE',  ( -3.996523416598930318E-16, 2.658563593772947863E-15, 1.000000000000000000 ) ) ;
#26870=ADVANCED_FACE ( 'NONE', ( #23585 ), #37061, .F. ) ;
#26899=ORIENTED_EDGE ( 'NONE', *, *, #5147, .T. ) ;
#26909=AXIS2_PLACEMENT_3D ( 'NONE', #33774, #4303, #40522 ) ;
#26981=VECTOR ( 'NONE', #7296, 1000.000000000000000 ) ;
#26998=EDGE_CURVE ( 'NONE', #24964, #29204, #23794, .T. ) ;
#27064=CARTESIAN_POINT ( 'NONE',  ( -2.797566391619251075E-15, 1.860994515641065082E-14, 7.000000000000002665 ) ) ;
#27073=CYLINDRICAL_SURFACE ( 'NONE', #38294, 19.99999999999989342 ) ;
#27104=ORIENTED_EDGE ( 'NONE', *, *, #19082, .T. ) ;
#27109=VERTEX_POINT ( 'NONE', #11549 ) ;
#27131=AXIS2_PLACEMENT_3D ( 'NONE', #19156, #12167, #25488 ) ;
#27182=DIRECTION ( 'NONE',  ( 1.000000000000000000, 0.000000000000000000, -6.546126324440847704E-16 ) ) ;
#27231=ORIENTED_EDGE ( 'NONE', *, *, #30523, .F. ) ;
#27249=DIRECTION ( 'NONE',  ( 1.000000000000000000, -1.373900992973641671E-15, -3.895519384649692070E-16 ) ) ;
#27275=DIRECTION ( 'NONE',  ( 1.000000000000000000, -1.373900992973643249E-15, -5.551115123125812284E-16 ) ) ;
#27289=ORIENTED_EDGE ( 'NONE', *, *, #37223, .T. ) ;
#27306=DIRECTION ( 'NONE',  ( 1.000000000000000000, 0.000000000000000000, -3.273063162220425331E-16 ) ) ;
#27344=FACE_OUTER_BOUND ( 'NONE', #32592, .T. ) ;
#27348=DIRECTION ( 'NONE',  ( -3.996523416598930318E-16, 2.658563593772947863E-15, 1.000000000000000000 ) ) ;
#27391=CARTESIAN_POINT ( 'NONE',  ( -1.420922472151883646E-13, 9.833206111663764869E-13, 369.6955262170047831 ) ) ;
#27398=VERTEX_POINT ( 'NONE', #23950 ) ;
#27473=FACE_BOUND ( 'NONE', #1807, .T. ) ;
#27506=VECTOR ( 'NONE', #4297, 1000.000000000000000 ) ;
#27521=DIRECTION ( 'NONE',  ( -3.996523416598930318E-16, 2.658563593772947863E-15, 1.000000000000000000 ) ) ;
#27692=CIRCLE ( 'NONE', #10961, 22.99999999999987921 ) ;
#27728=DIRECTION ( 'NONE',  ( -3.996523416598930318E-16, 2.658563593772947863E-15, 1.000000000000000000 ) ) ;
#27740=EDGE_CURVE ( 'NONE', #8724, #25091, #30343, .T. ) ;
#27780=CARTESIAN_POINT ( 'NONE',  ( 103.7695705685756877, -106.4195705685758213, 6.999999999999666933 ) ) ;
#27807=ORIENTED_EDGE ( 'NONE', *, *, #25527, .T. ) ;
#27902=CARTESIAN_POINT ( 'NONE',  ( -109.0695705685741785, -106.4195705685773135, 9.999999999999751310 ) ) ;
#27909=DIRECTION ( 'NONE',  ( 1.000000000000000000, 0.000000000000000000, -3.273063162220425331E-16 ) ) ;
#27960=CARTESIAN_POINT ( 'NONE',  ( 142.4999999999992895, -3.154162532185255727E-13, -45.00000000000004974 ) ) ;
#28039=PLANE ( 'NONE',  #15077 ) ;
#28047=DIRECTION ( 'NONE',  ( 0.2140725878556618555, -0.9768177553304301375, -2.795573601670286284E-15 ) ) ;
#28061=DIRECTION ( 'NONE',  ( -3.996523416598930318E-16, 2.658563593772947863E-15, 1.000000000000000000 ) ) ;
#28069=DIRECTION ( 'NONE',  ( -3.996523416598930318E-16, 2.658563593772947863E-15, 1.000000000000000000 ) ) ;
#28105=ORIENTED_EDGE ( 'NONE', *, *, #33012, .F. ) ;
#28109=CARTESIAN_POINT ( 'NONE',  ( -106.4195705685741871, -106.4195705685773135, 6.999999999999754863 ) ) ;
#28122=CARTESIAN_POINT ( 'NONE',  ( 130.0000000000000000, -2.127378845942280309E-13, 2.000000000000031530 ) ) ;
#28153=DIRECTION ( 'NONE',  ( 1.000000000000000000, -1.373900992973643249E-15, -5.551115123125812284E-16 ) ) ;
#28181=EDGE_CURVE ( 'NONE', #23479, #13925, #28314, .T. ) ;
#28187=DIRECTION ( 'NONE',  ( 1.000000000000000000, -1.373900992973641868E-15, -6.546126324440886161E-16 ) ) ;
#28228=EDGE_LOOP ( 'NONE', ( #34350, #15683 ) ) ;
#28239=ORIENTED_EDGE ( 'NONE', *, *, #14242, .T. ) ;
#28261=ORIENTED_EDGE ( 'NONE', *, *, #30523, .T. ) ;
#28314=CIRCLE ( 'NONE', #17862, 139.4999999999992610 ) ;
#28326=ORIENTED_EDGE ( 'NONE', *, *, #10848, .F. ) ;
#28334=EDGE_CURVE ( 'NONE', #19047, #35963, #24840, .T. ) ;
#28359=VERTEX_POINT ( 'NONE', #33795 ) ;
#28374=DIRECTION ( 'NONE',  ( -3.996523416598930318E-16, 2.658563593772947863E-15, 1.000000000000000000 ) ) ;
#28408=AXIS2_PLACEMENT_3D ( 'NONE', #74, #14297, #10137 ) ;
#28430=EDGE_LOOP ( 'NONE', ( #33909, #20048, #32223, #16342 ) ) ;
#28435=ORIENTED_EDGE ( 'NONE', *, *, #30450, .F. ) ;
#28436=AXIS2_PLACEMENT_3D ( 'NONE', #22801, #23016, #18900 ) ;
#28485=FACE_BOUND ( 'NONE', #1092, .T. ) ;
#28501=AXIS2_PLACEMENT_3D ( 'NONE', #19518, #10082, #13387 ) ;
#28503=CARTESIAN_POINT ( 'NONE',  ( 1.798435537469519230E-14, -1.196353617197826191E-13, -44.99999999999999289 ) ) ;
#28527=DIRECTION ( 'NONE',  ( -3.996523416598930318E-16, 2.658563593772947863E-15, 1.000000000000000000 ) ) ;
#28554=CARTESIAN_POINT ( 'NONE',  ( 1.798435537469519230E-14, -1.196353617197826191E-13, -44.99999999999999289 ) ) ;
#28559=DIRECTION ( 'NONE',  ( 1.000000000000000000, 0.000000000000000000, -6.546126324440850663E-16 ) ) ;
#28574=CIRCLE ( 'NONE', #16045, 158.4999999999992042 ) ;
#28582=LINE ( 'NONE', #11559, #30562 ) ;
#28587=LINE ( 'NONE', #8698, #2087 ) ;
#28601=VERTEX_POINT ( 'NONE', #2967 ) ;
#28625=AXIS2_PLACEMENT_3D ( 'NONE', #10381, #20238, #33499 ) ;
#28644=EDGE_LOOP ( 'NONE', ( #9525, #42222 ) ) ;
#28740=EDGE_LOOP ( 'NONE', ( #27104, #11783, #28988, #15412 ) ) ;
#28757=CYLINDRICAL_SURFACE ( 'NONE', #33833, 139.4999999999992610 ) ;
#28815=CYLINDRICAL_SURFACE ( 'NONE', #36286, 129.9999999999993463 ) ;
#28872=PRESENTATION_STYLE_ASSIGNMENT (( #2216 ) ) ;
#28897=DIRECTION ( 'NONE',  ( 1.000000000000000000, 0.000000000000000000, -3.273063162220425331E-16 ) ) ;
#28988=ORIENTED_EDGE ( 'NONE', *, *, #15390, .T. ) ;
#29046=ORIENTED_EDGE ( 'NONE', *, *, #18809, .T. ) ;
#29058=PRODUCT ( 'housing right', 'housing right', '', ( #21458 ) ) ;
#29148=DIRECTION ( 'NONE',  ( 1.000000000000000000, -1.373900992973641868E-15, -3.469446951953632924E-16 ) ) ;
#29194=VERTEX_POINT ( 'NONE', #30446 ) ;
#29204=VERTEX_POINT ( 'NONE', #7517 ) ;
#29220=DIRECTION ( 'NONE',  ( -3.996523416598930318E-16, 2.658563593772947863E-15, 1.000000000000000000 ) ) ;
#29230=EDGE_CURVE ( 'NONE', #23893, #27109, #1201, .T. ) ;
#29231=ORIENTED_EDGE ( 'NONE', *, *, #21891, .T. ) ;
#29241=ORIENTED_EDGE ( 'NONE', *, *, #9323, .T. ) ;
#29334=DIRECTION ( 'NONE',  ( -3.996523416598930318E-16, 2.658563593772947863E-15, 1.000000000000000000 ) ) ;
#29423=VECTOR ( 'NONE', #1523, 1000.000000000000000 ) ;
#29431=FACE_BOUND ( 'NONE', #34111, .T. ) ;
#29439=ADVANCED_FACE ( 'NONE', ( #19310 ), #5743, .F. ) ;
#29472=CARTESIAN_POINT ( 'NONE',  ( -2.095696658341510008E-13, 150.5000000000013642, 7.000000000000419220 ) ) ;
#29499=CARTESIAN_POINT ( 'NONE',  ( -2.797566391619251075E-15, 1.860994515641065082E-14, 7.000000000000002665 ) ) ;
#29501=AXIS2_PLACEMENT_3D ( 'NONE', #21977, #2478, #29148 ) ;
#29519=ADVANCED_FACE ( 'NONE', ( #29528 ), #32363, .T. ) ;
#29528=FACE_OUTER_BOUND ( 'NONE', #2714, .T. ) ;
#29531=ADVANCED_FACE ( 'NONE', ( #25647, #38905 ), #9023, .T. ) ;
#29604=VERTEX_POINT ( 'NONE', #3722 ) ;
#29643=VERTEX_POINT ( 'NONE', #14247 ) ;
#29780=CARTESIAN_POINT ( 'NONE',  ( -2.841217984690893843E-16, 1.478917074864463474E-14, 1.999999999999980904 ) ) ;
#29818=AXIS2_PLACEMENT_3D ( 'NONE', #16837, #29916, #23367 ) ;
#29870=ADVANCED_FACE ( 'NONE', ( #42334 ), #12900, .T. ) ;
#29876=ORIENTED_EDGE ( 'NONE', *, *, #28334, .T. ) ;
#29916=DIRECTION ( 'NONE',  ( -3.996523416598930318E-16, 2.658563593772947863E-15, 1.000000000000000000 ) ) ;
#29944=EDGE_CURVE ( 'NONE', #27398, #22603, #25702, .T. ) ;
#29950=FACE_OUTER_BOUND ( 'NONE', #24767, .T. ) ;
#29965=DIRECTION ( 'NONE',  ( 1.000000000000000000, 0.000000000000000000, -6.546126324440850663E-16 ) ) ;
#29980=EDGE_LOOP ( 'NONE', ( #39852, #33330, #30298, #4136 ) ) ;
#30063=ORIENTED_EDGE ( 'NONE', *, *, #10507, .T. ) ;
#30109=DIRECTION ( 'NONE',  ( -3.996523416598930318E-16, 2.658563593772947863E-15, 1.000000000000000000 ) ) ;
#30140=CARTESIAN_POINT ( 'NONE',  ( 158.4999999999992042, -1.991533622299105221E-13, 6.999999999999939604 ) ) ;
#30160=DIRECTION ( 'NONE',  ( -3.996523416598930318E-16, 2.658563593772947863E-15, 1.000000000000000000 ) ) ;
#30193=EDGE_CURVE ( 'NONE', #6244, #29643, #35682, .T. ) ;
#30196=VECTOR ( 'NONE', #41336, 1000.000000000000000 ) ;
#30298=ORIENTED_EDGE ( 'NONE', *, *, #7651, .T. ) ;
#30343=CIRCLE ( 'NONE', #38669, 22.99999999999987921 ) ;
#30394=ORIENTED_EDGE ( 'NONE', *, *, #9828, .T. ) ;
#30403=DIRECTION ( 'NONE',  ( -3.996523416598930318E-16, 2.658563593772947863E-15, 1.000000000000000000 ) ) ;
#30405=ORIENTED_EDGE ( 'NONE', *, *, #10848, .T. ) ;
#30446=CARTESIAN_POINT ( 'NONE',  ( -2.650000000000198419, 150.5000000000013642, 10.00000000000041744 ) ) ;
#30450=EDGE_CURVE ( 'NONE', #34755, #2151, #26111, .T. ) ;
#30468=EDGE_CURVE ( 'NONE', #24680, #239, #23611, .T. ) ;
#30523=EDGE_CURVE ( 'NONE', #23479, #3549, #14536, .T. ) ;
#30544=FACE_BOUND ( 'NONE', #39865, .T. ) ;
#30551=EDGE_CURVE ( 'NONE', #20249, #38954, #40216, .T. ) ;
#30562=VECTOR ( 'NONE', #22476, 1000.000000000000000 ) ;
#30571=EDGE_LOOP ( 'NONE', ( #42798, #19432, #23657, #40291 ) ) ;
#30576=LINE ( 'NONE', #30140, #36213 ) ;
#30618=DIRECTION ( 'NONE',  ( -3.892440008040322386E-16, 2.658563593772947863E-15, 1.000000000000000000 ) ) ;
#30633=ADVANCED_FACE ( 'NONE', ( #18703 ), #31965, .T. ) ;
#30660=ORIENTED_EDGE ( 'NONE', *, *, #1705, .F. ) ;
#30669=AXIS2_PLACEMENT_3D ( 'NONE', #28554, #4747, #18114 ) ;
#30742=ORIENTED_EDGE ( 'NONE', *, *, #25641, .T. ) ;
#30778=EDGE_LOOP ( 'NONE', ( #35219, #21011, #24703, #18127 ) ) ;
#30821=AXIS2_PLACEMENT_3D ( 'NONE', #25588, #32102, #8531 ) ;
#30826=ORIENTED_EDGE ( 'NONE', *, *, #38162, .F. ) ;
#30868=DIRECTION ( 'NONE',  ( -3.996523416598930318E-16, 2.658563593772947863E-15, 1.000000000000000000 ) ) ;
#30951=DIRECTION ( 'NONE',  ( 1.000000000000000000, -1.373900992973641868E-15, -3.273063162220443081E-16 ) ) ;
#31000=ADVANCED_FACE ( 'NONE', ( #27344 ), #6826, .F. ) ;
#31029=EDGE_LOOP ( 'NONE', ( #38481, #30394 ) ) ;
#31038=ORIENTED_EDGE ( 'NONE', *, *, #36760, .T. ) ;
#31089=MECHANICAL_DESIGN_GEOMETRIC_PRESENTATION_REPRESENTATION('',(#20652),#17892);
#31090=EDGE_CURVE ( 'NONE', #29643, #42975, #17031, .T. ) ;
#31108=EDGE_CURVE ( 'NONE', #17574, #29604, #5129, .T. ) ;
#31175=ORIENTED_EDGE ( 'NONE', *, *, #26316, .T. ) ;
#31186=FACE_BOUND ( 'NONE', #32594, .T. ) ;
#31204=FACE_OUTER_BOUND ( 'NONE', #18670, .T. ) ;
#31253=AXIS2_PLACEMENT_3D ( 'NONE', #32734, #22966, #2817 ) ;
#31256=VERTEX_POINT ( 'NONE', #17503 ) ;
#31276=AXIS2_PLACEMENT_3D ( 'NONE', #20880, #24359, #28047 ) ;
#31318=CARTESIAN_POINT ( 'NONE',  ( 104.9999999999993321, -2.293336392629658115E-13, -32.00000000000000000 ) ) ;
#31340=CARTESIAN_POINT ( 'NONE',  ( 2.027755760259328333E-13, -150.5000000000013642, 9.999999999999586109 ) ) ;
#31355=ORIENTED_EDGE ( 'NONE', *, *, #23394, .T. ) ;
#31416=CARTESIAN_POINT ( 'NONE',  ( 2.649999999999762323, 150.5000000000013642, 10.00000000000041744 ) ) ;
#31440=CARTESIAN_POINT ( 'NONE',  ( 147.8499999999987438, 1.400182730016050856E-12, 9.999999999999962697 ) ) ;
#31515=FACE_BOUND ( 'NONE', #31029, .T. ) ;
#31583=FACE_OUTER_BOUND ( 'NONE', #22746, .T. ) ;
#31587=FACE_OUTER_BOUND ( 'NONE', #23455, .T. ) ;
#31597=CARTESIAN_POINT ( 'NONE',  ( 102.9999999999993463, -2.265858372770185743E-13, -32.00000000000000000 ) ) ;
#31600=EDGE_CURVE ( 'NONE', #28601, #5117, #10880, .T. ) ;
#31631=( GEOMETRIC_REPRESENTATION_CONTEXT ( 3 ) GLOBAL_UNCERTAINTY_ASSIGNED_CONTEXT ( ( #38599 ) ) GLOBAL_UNIT_ASSIGNED_CONTEXT ( ( #18440, #18671, #4870 ) ) REPRESENTATION_CONTEXT ( 'NONE', 'WORKASPACE' ) );
#31707=EDGE_CURVE ( 'NONE', #11569, #25432, #24214, .T. ) ;
#31722=CARTESIAN_POINT ( 'NONE',  ( 20.00000000000001776, -1.127613248556852545E-13, -39.99999999999999289 ) ) ;
#31724=FACE_BOUND ( 'NONE', #19696, .T. ) ;
#31734=CIRCLE ( 'NONE', #5922, 2.649999999999973266 ) ;
#31742=DIRECTION ( 'NONE',  ( 3.996523416598930318E-16, -2.658563593772947863E-15, -1.000000000000000000 ) ) ;
#31766=DIRECTION ( 'NONE',  ( 1.000000000000000000, 0.000000000000000000, -6.546126324440850663E-16 ) ) ;
#31847=DIRECTION ( 'NONE',  ( 1.000000000000000000, 0.000000000000000000, -6.546126324440850663E-16 ) ) ;
#31870=DIRECTION ( 'NONE',  ( -1.000000000000000000, 1.373900992973641671E-15, 4.270088556250623393E-16 ) ) ;
#31884=CYLINDRICAL_SURFACE ( 'NONE', #35972, 2.649999999999957723 ) ;
#31889=DIRECTION ( 'NONE',  ( 1.000000000000000000, -1.373900992973642263E-15, -3.016910393003158636E-16 ) ) ;
#31923=CIRCLE ( 'NONE', #11765, 1.999999999999988010 ) ;
#31929=EDGE_LOOP ( 'NONE', ( #8203, #31355, #43091, #21934 ) ) ;
#31931=PRESENTATION_STYLE_ASSIGNMENT (( #1804 ) ) ;
#31960=ADVANCED_FACE ( 'NONE', ( #39814 ), #2731, .F. ) ;
#31965=CYLINDRICAL_SURFACE ( 'NONE', #10271, 1.999999999999988010 ) ;
#32018=EDGE_CURVE ( 'NONE', #40947, #239, #36543, .T. ) ;
#32019=CYLINDRICAL_SURFACE ( 'NONE', #30669, 142.4999999999992610 ) ;
#32023=CARTESIAN_POINT ( 'NONE',  ( -106.4195705685741871, -106.4195705685773135, 9.999999999999751310 ) ) ;
#32056=ORIENTED_EDGE ( 'NONE', *, *, #35907, .F. ) ;
#32100=AXIS2_PLACEMENT_3D ( 'NONE', #32260, #29220, #38796 ) ;
#32102=DIRECTION ( 'NONE',  ( 3.996523416598930318E-16, -2.658563593772947863E-15, -1.000000000000000000 ) ) ;
#32127=FACE_OUTER_BOUND ( 'NONE', #25643, .T. ) ;
#32177=LINE ( 'NONE', #17360, #35322 ) ;
#32182=AXIS2_PLACEMENT_3D ( 'NONE', #17304, #13147, #6992 ) ;
#32183=DIRECTION ( 'NONE',  ( 1.000000000000000000, 0.000000000000000000, -6.546126324440832913E-16 ) ) ;
#32223=ORIENTED_EDGE ( 'NONE', *, *, #27740, .T. ) ;
#32260=CARTESIAN_POINT ( 'NONE',  ( -106.4195705685749402, 106.4195705685765745, 10.00000000000033751 ) ) ;
#32265=DIRECTION ( 'NONE',  ( -3.996523416598930318E-16, 2.658563593772947863E-15, 1.000000000000000000 ) ) ;
#32279=VERTEX_POINT ( 'NONE', #19061 ) ;
#32309=DIRECTION ( 'NONE',  ( -1.000000000000000000, 1.373900992973642263E-15, 0.000000000000000000 ) ) ;
#32363=CYLINDRICAL_SURFACE ( 'NONE', #10276, 22.99999999999987921 ) ;
#32380=DIRECTION ( 'NONE',  ( 1.000000000000000000, -1.373900992973641868E-15, -6.546126324440886161E-16 ) ) ;
#32384=AXIS2_PLACEMENT_3D ( 'NONE', #9017, #26465, #27275 ) ;
#32386=DIRECTION ( 'NONE',  ( -3.996523416598930318E-16, 2.658563593772947863E-15, 1.000000000000000000 ) ) ;
#32390=DIRECTION ( 'NONE',  ( 1.000000000000000000, 0.000000000000000000, -3.273063162220416457E-16 ) ) ;
#32464=VERTEX_POINT ( 'NONE', #16200 ) ;
#32525=EDGE_LOOP ( 'NONE', ( #7932, #9745 ) ) ;
#32559=CIRCLE ( 'NONE', #10969, 2.649999999999971934 ) ;
#32592=EDGE_LOOP ( 'NONE', ( #19868, #7001, #16848, #26026 ) ) ;
#32594=EDGE_LOOP ( 'NONE', ( #42822, #35956 ) ) ;
#32611=ORIENTED_EDGE ( 'NONE', *, *, #31108, .T. ) ;
#32678=CARTESIAN_POINT ( 'NONE',  ( -106.4195705685741871, -106.4195705685773135, 9.999999999999751310 ) ) ;
#32702=DIRECTION ( 'NONE',  ( -3.996523416598930318E-16, 2.658563593772947863E-15, 1.000000000000000000 ) ) ;
#32734=CARTESIAN_POINT ( 'NONE',  ( -2.095696658341510008E-13, 150.5000000000013642, 7.000000000000419220 ) ) ;
#32735=AXIS2_PLACEMENT_3D ( 'NONE', #4942, #4488, #17865 ) ;
#32736=ORIENTED_EDGE ( 'NONE', *, *, #1705, .T. ) ;
#32776=VERTEX_POINT ( 'NONE', #12026 ) ;
#32827=APPLICATION_CONTEXT ( 'automotive_design' ) ;
#32939=DIRECTION ( 'NONE',  ( 1.000000000000000000, 0.000000000000000000, -3.273063162220416457E-16 ) ) ;
#32948=CARTESIAN_POINT ( 'NONE',  ( -2.797566391619251075E-15, 1.860994515641065082E-14, 7.000000000000002665 ) ) ;
#32971=VERTEX_POINT ( 'NONE', #36609 ) ;
#33006=EDGE_LOOP ( 'NONE', ( #40383, #38488 ) ) ;
#33011=EDGE_CURVE ( 'NONE', #15772, #17775, #15103, .T. ) ;
#33012=EDGE_CURVE ( 'NONE', #39874, #31256, #39430, .T. ) ;
#33028=DIRECTION ( 'NONE',  ( -1.000000000000000000, 1.373900992973641868E-15, 4.405646923115722869E-16 ) ) ;
#33052=DIRECTION ( 'NONE',  ( -3.996523416598930318E-16, 2.658563593772947863E-15, 1.000000000000000000 ) ) ;
#33064=EDGE_CURVE ( 'NONE', #14258, #25432, #10877, .T. ) ;
#33149=AXIS2_PLACEMENT_3D ( 'NONE', #29780, #48, #36290 ) ;
#33188=FACE_OUTER_BOUND ( 'NONE', #20180, .T. ) ;
#33192=CIRCLE ( 'NONE', #40840, 22.99999999999987921 ) ;
#33217=LINE ( 'NONE', #14188, #23353 ) ;
#33300=DIRECTION ( 'NONE',  ( 3.996523416598930318E-16, -2.658563593772947863E-15, -1.000000000000000000 ) ) ;
#33330=ORIENTED_EDGE ( 'NONE', *, *, #21702, .F. ) ;
#33389=DIRECTION ( 'NONE',  ( -3.996523416598930318E-16, 2.658563593772947863E-15, 1.000000000000000000 ) ) ;
#33407=CARTESIAN_POINT ( 'NONE',  ( -103.7695705685742240, -106.4195705685773135, 6.999999999999753975 ) ) ;
#33408=EDGE_CURVE ( 'NONE', #25656, #26054, #19995, .T. ) ;
#33443=CARTESIAN_POINT ( 'NONE',  ( -2.107686228591307694E-13, 150.5000000000013642, 10.00000000000041744 ) ) ;
#33451=CARTESIAN_POINT ( 'NONE',  ( 150.4999999999986926, 1.388241670201576064E-12, 6.999999999999959144 ) ) ;
#33460=AXIS2_PLACEMENT_3D ( 'NONE', #41417, #2138, #18360 ) ;
#33499=DIRECTION ( 'NONE',  ( 1.000000000000000000, 0.000000000000000000, -3.273063162220425331E-16 ) ) ;
#33554=CARTESIAN_POINT ( 'NONE',  ( -1.420922472151883646E-13, 9.833206111663764869E-13, 369.6955262170047831 ) ) ;
#33565=ORIENTED_EDGE ( 'NONE', *, *, #30551, .F. ) ;
#33575=DIRECTION ( 'NONE',  ( 1.000000000000000000, 0.000000000000000000, -6.546126324440850663E-16 ) ) ;
#33612=CYLINDRICAL_SURFACE ( 'NONE', #32182, 2.649999999999971934 ) ;
#33624=EDGE_CURVE ( 'NONE', #21317, #2151, #40863, .T. ) ;
#33635=VECTOR ( 'NONE', #6239, 1000.000000000000000 ) ;
#33653=DIRECTION ( 'NONE',  ( 1.000000000000000000, -1.373900992973642263E-15, -3.996523416598957436E-16 ) ) ;
#33696=CARTESIAN_POINT ( 'NONE',  ( 109.0695705685734254, 106.4195705685780524, 10.00000000000025047 ) ) ;
#33701=( GEOMETRIC_REPRESENTATION_CONTEXT ( 3 ) GLOBAL_UNCERTAINTY_ASSIGNED_CONTEXT ( ( #17835 ) ) GLOBAL_UNIT_ASSIGNED_CONTEXT ( ( #25202, #41935, #15573 ) ) REPRESENTATION_CONTEXT ( 'NONE', 'WORKASPACE' ) );
#33707=VECTOR ( 'NONE', #20506, 1000.000000000000000 ) ;
#33774=CARTESIAN_POINT ( 'NONE',  ( 1.598609366639573350E-14, -1.063425437509180407E-13, -40.00000000000000000 ) ) ;
#33786=EDGE_LOOP ( 'NONE', ( #12856, #17559, #21723, #16243 ) ) ;
#33795=CARTESIAN_POINT ( 'NONE',  ( 153.1499999999986414, 1.384600832570195860E-12, 6.999999999999958256 ) ) ;
#33829=EDGE_LOOP ( 'NONE', ( #17605, #17215 ) ) ;
#33833=AXIS2_PLACEMENT_3D ( 'NONE', #34633, #8658, #4513 ) ;
#33858=EDGE_CURVE ( 'NONE', #25656, #32464, #16480, .T. ) ;
#33861=EDGE_CURVE ( 'NONE', #40947, #41484, #15769, .T. ) ;
#33908=AXIS2_PLACEMENT_3D ( 'NONE', #42787, #26251, #39098 ) ;
#33909=ORIENTED_EDGE ( 'NONE', *, *, #2057, .F. ) ;
#33976=CARTESIAN_POINT ( 'NONE',  ( -2.649999999999789857, -150.5000000000013642, 6.999999999999585221 ) ) ;
#34094=DIRECTION ( 'NONE',  ( 1.000000000000000000, 0.000000000000000000, -6.546126324440850663E-16 ) ) ;
#34111=EDGE_LOOP ( 'NONE', ( #32056, #28105 ) ) ;
#34199=FACE_OUTER_BOUND ( 'NONE', #31929, .T. ) ;
#34201=CARTESIAN_POINT ( 'NONE',  ( 103.7695705685757019, -106.4195705685758213, 9.999999999999671374 ) ) ;
#34205=DIRECTION ( 'NONE',  ( -3.996523416598930318E-16, 2.658563593772947863E-15, 1.000000000000000000 ) ) ;
#34264=CARTESIAN_POINT ( 'NONE',  ( 106.4195705685734623, 106.4195705685780524, 7.000000000000250466 ) ) ;
#34307=ORIENTED_EDGE ( 'NONE', *, *, #38521, .F. ) ;
#34322=CIRCLE ( 'NONE', #14862, 2.649999999999957723 ) ;
#34350=ORIENTED_EDGE ( 'NONE', *, *, #30468, .F. ) ;
#34370=VERTEX_POINT ( 'NONE', #43164 ) ;
#34386=CYLINDRICAL_SURFACE ( 'NONE', #32735, 142.4999999999992610 ) ;
#34424=DIRECTION ( 'NONE',  ( 3.996523416598930318E-16, -2.658563593772947863E-15, -1.000000000000000000 ) ) ;
#34441=DIRECTION ( 'NONE',  ( -3.996523416598930318E-16, 2.658563593772947863E-15, 1.000000000000000000 ) ) ;
#34574=DIRECTION ( 'NONE',  ( 1.000000000000000000, -1.373900992973642263E-15, -3.996523416598957436E-16 ) ) ;
#34633=CARTESIAN_POINT ( 'NONE',  ( -3.996523416598931009E-15, 2.658563593772952281E-14, 10.00000000000000178 ) ) ;
#34643=DIRECTION ( 'NONE',  ( 1.000000000000000000, -1.373900992973642263E-15, 0.000000000000000000 ) ) ;
#34655=FACE_BOUND ( 'NONE', #3839, .T. ) ;
#34698=EDGE_LOOP ( 'NONE', ( #5803, #39118 ) ) ;
#34699=LINE ( 'NONE', #31440, #29423 ) ;
#34755=VERTEX_POINT ( 'NONE', #33976 ) ;
#34775=DIRECTION ( 'NONE',  ( 3.996523416598993920E-16, 2.658563593772947074E-15, 1.000000000000000000 ) ) ;
#34895=CIRCLE ( 'NONE', #16012, 2.649999999999971934 ) ;
#34923=CIRCLE ( 'NONE', #1460, 2.649999999999957723 ) ;
#34926=CARTESIAN_POINT ( 'NONE',  ( 150.4999999999986926, 1.396217360982896810E-12, 9.999999999999960920 ) ) ;
#35005=PLANE ( 'NONE',  #20872 ) ;
#35017=AXIS2_PLACEMENT_3D ( 'NONE', #32678, #10412, #3410 ) ;
#35056=DIRECTION ( 'NONE',  ( -3.996523416598930318E-16, 2.658563593772947863E-15, 1.000000000000000000 ) ) ;
#35128=CIRCLE ( 'NONE', #14226, 2.649999999999971934 ) ;
#35139=EDGE_CURVE ( 'NONE', #9697, #36354, #32559, .T. ) ;
#35141=CARTESIAN_POINT ( 'NONE',  ( 150.4999999999986926, 1.396217360982896810E-12, 9.999999999999962697 ) ) ;
#35184=EDGE_LOOP ( 'NONE', ( #5854, #36363, #7836, #40889 ) ) ;
#35189=EDGE_CURVE ( 'NONE', #20926, #9697, #43084, .T. ) ;
#35218=AXIS2_PLACEMENT_3D ( 'NONE', #39402, #16314, #43115 ) ;
#35219=ORIENTED_EDGE ( 'NONE', *, *, #22114, .F. ) ;
#35227=DIRECTION ( 'NONE',  ( 1.000000000000000000, 0.000000000000000000, -6.546126324440847704E-16 ) ) ;
#35238=AXIS2_PLACEMENT_3D ( 'NONE', #10889, #1261, #34643 ) ;
#35252=VECTOR ( 'NONE', #7241, 1000.000000000000000 ) ;
#35307=ORIENTED_EDGE ( 'NONE', *, *, #18377, .T. ) ;
#35308=CIRCLE ( 'NONE', #20718, 22.99999999999987921 ) ;
#35322=VECTOR ( 'NONE', #40851, 1000.000000000000000 ) ;
#35389=EDGE_CURVE ( 'NONE', #23944, #18098, #19401, .T. ) ;
#35392=CARTESIAN_POINT ( 'NONE',  ( -106.4195705685741871, -106.4195705685773135, 9.999999999999753086 ) ) ;
#35417=CARTESIAN_POINT ( 'NONE',  ( -3.996523416598931009E-15, 2.658563593772952281E-14, 10.00000000000000178 ) ) ;
#35447=DIRECTION ( 'NONE',  ( -3.996523416598930318E-16, 2.658563593772947863E-15, 1.000000000000000000 ) ) ;
#35543=CARTESIAN_POINT ( 'NONE',  ( -1.420922472151883646E-13, 9.833206111663764869E-13, 369.6955262170047831 ) ) ;
#35588=DIRECTION ( 'NONE',  ( 1.000000000000000000, 0.000000000000000000, -6.546126324440850663E-16 ) ) ;
#35603=CYLINDRICAL_SURFACE ( 'NONE', #20604, 2.649999999999957723 ) ;
#35635=FACE_OUTER_BOUND ( 'NONE', #20826, .T. ) ;
#35682=LINE ( 'NONE', #5595, #4775 ) ;
#35686=CARTESIAN_POINT ( 'NONE',  ( 12.49999999999995204, -1.368091241319530598E-13, -45.00000000000000000 ) ) ;
#35730=DIRECTION ( 'NONE',  ( 1.000000000000000000, -1.373900992973641868E-15, -4.017254365419995317E-16 ) ) ;
#35754=AXIS2_PLACEMENT_3D ( 'NONE', #22405, #19128, #32183 ) ;
#35768=DIRECTION ( 'NONE',  ( 3.996523416598930318E-16, -2.658563593772947863E-15, -1.000000000000000000 ) ) ;
#35804=CLOSED_SHELL ( 'NONE', ( #29870, #11295, #3794, #40196, #13325, #10875, #3634, #18656, #31000, #41480, #4086, #3024, #8423, #19867, #24373, #16560, #38991, #11983, #37008, #7923, #13795, #36700, #31960, #14009, #29519, #36851, #40491, #43171, #29531, #6312, #7718, #24661, #12434, #26307, #26870, #20355, #11803, #26145, #20598, #3459, #29439, #30633, #1539 ) ) ;
#35848=CIRCLE ( 'NONE', #32384, 12.49999999999993427 ) ;
#35887=EDGE_LOOP ( 'NONE', ( #3754, #30405 ) ) ;
#35907=EDGE_CURVE ( 'NONE', #31256, #39874, #31923, .T. ) ;
#35908=EDGE_CURVE ( 'NONE', #37599, #37475, #25597, .T. ) ;
#35909=DIRECTION ( 'NONE',  ( -3.996523416598930318E-16, 2.658563593772947863E-15, 1.000000000000000000 ) ) ;
#35911=ORIENTED_EDGE ( 'NONE', *, *, #8607, .F. ) ;
#35928=CARTESIAN_POINT ( 'NONE',  ( 1.598609366639573350E-14, -1.063425437509180407E-13, -40.00000000000000000 ) ) ;
#35946=COLOUR_RGB ( '', 0.31764706, 0.68627451, 0.89019608) ;
#35956=ORIENTED_EDGE ( 'NONE', *, *, #18406, .F. ) ;
#35963=VERTEX_POINT ( 'NONE', #22327 ) ;
#35970=ORIENTED_EDGE ( 'NONE', *, *, #35907, .T. ) ;
#35972=AXIS2_PLACEMENT_3D ( 'NONE', #34926, #5038, #28187 ) ;
#36129=EDGE_CURVE ( 'NONE', #5117, #37475, #36820, .T. ) ;
#36174=AXIS2_PLACEMENT_3D ( 'NONE', #14832, #37272, #23793 ) ;
#36178=DIRECTION ( 'NONE',  ( 1.000000000000000000, -1.373900992973641868E-15, -3.273063162220443081E-16 ) ) ;
#36213=VECTOR ( 'NONE', #196, 1000.000000000000000 ) ;
#36242=EDGE_LOOP ( 'NONE', ( #15506, #16616, #25010, #39994 ) ) ;
#36286=AXIS2_PLACEMENT_3D ( 'NONE', #35543, #18603, #31870 ) ;
#36290=DIRECTION ( 'NONE',  ( 0.2140725878556618555, -0.9768177553304301375, -2.795573601670286284E-15 ) ) ;
#36311=LINE ( 'NONE', #19780, #10245 ) ;
#36340=DIRECTION ( 'NONE',  ( 1.000000000000000000, -1.373900992973641277E-15, -5.551115123125812284E-16 ) ) ;
#36354=VERTEX_POINT ( 'NONE', #20545 ) ;
#36363=ORIENTED_EDGE ( 'NONE', *, *, #31600, .T. ) ;
#36497=EDGE_CURVE ( 'NONE', #16254, #36354, #23923, .T. ) ;
#36499=EDGE_LOOP ( 'NONE', ( #15437, #5678, #24688, #11146 ) ) ;
#36543=LINE ( 'NONE', #9088, #20551 ) ;
#36549=CARTESIAN_POINT ( 'NONE',  ( 1.798435537469519230E-14, -1.196353617197826191E-13, -44.99999999999999289 ) ) ;
#36568=EDGE_LOOP ( 'NONE', ( #28435, #42217, #39136, #7038 ) ) ;
#36609=CARTESIAN_POINT ( 'NONE',  ( 20.00000000000001066, -1.127613248556854817E-13, -25.99999999999999645 ) ) ;
#36700=ADVANCED_FACE ( 'NONE', ( #5113, #41099 ), #35005, .F. ) ;
#36757=VECTOR ( 'NONE', #43176, 1000.000000000000000 ) ;
#36760=EDGE_CURVE ( 'NONE', #35963, #23893, #37623, .T. ) ;
#36817=FACE_OUTER_BOUND ( 'NONE', #30571, .T. ) ;
#36820=CIRCLE ( 'NONE', #24327, 142.4999999999992610 ) ;
#36851=ADVANCED_FACE ( 'NONE', ( #35635 ), #2673, .F. ) ;
#37006=EDGE_CURVE ( 'NONE', #28359, #19368, #23008, .T. ) ;
#37008=ADVANCED_FACE ( 'NONE', ( #43039, #13192 ), #17117, .T. ) ;
#37061=CYLINDRICAL_SURFACE ( 'NONE', #5846, 2.649999999999971934 ) ;
#37077=CARTESIAN_POINT ( 'NONE',  ( -109.0695705685741643, -106.4195705685773135, 9.999999999999753086 ) ) ;
#37096=DIRECTION ( 'NONE',  ( 1.000000000000000000, -1.373900992973641868E-15, -3.994789077170585140E-16 ) ) ;
#37119=VECTOR ( 'NONE', #21401, 1000.000000000000000 ) ;
#37187=DIRECTION ( 'NONE',  ( -3.996523416598930318E-16, 2.658563593772947863E-15, 1.000000000000000000 ) ) ;
#37223=EDGE_CURVE ( 'NONE', #4344, #32776, #21654, .T. ) ;
#37236=VECTOR ( 'NONE', #30109, 1000.000000000000000 ) ;
#37272=DIRECTION ( 'NONE',  ( 3.996523416598993920E-16, 2.658563593772947074E-15, 1.000000000000000000 ) ) ;
#37291=CIRCLE ( 'NONE', #10133, 139.4999999999992610 ) ;
#37431=CARTESIAN_POINT ( 'NONE',  ( 12.49999999999995204, -1.368091241319530598E-13, -45.00000000000000000 ) ) ;
#37432=DIRECTION ( 'NONE',  ( -3.996523416598930318E-16, 2.658563593772947863E-15, 1.000000000000000000 ) ) ;
#37465=EDGE_CURVE ( 'NONE', #19047, #27109, #30576, .T. ) ;
#37468=CIRCLE ( 'NONE', #20079, 142.4999999999992610 ) ;
#37472=ORIENTED_EDGE ( 'NONE', *, *, #40367, .T. ) ;
#37475=VERTEX_POINT ( 'NONE', #9831 ) ;
#37483=DIRECTION ( 'NONE',  ( -3.996523416598930318E-16, 2.658563593772947863E-15, 1.000000000000000000 ) ) ;
#37497=FACE_OUTER_BOUND ( 'NONE', #3662, .T. ) ;
#37511=AXIS2_PLACEMENT_3D ( 'NONE', #6926, #26159, #19426 ) ;
#37530=ORIENTED_EDGE ( 'NONE', *, *, #9749, .F. ) ;
#37573=DIRECTION ( 'NONE',  ( 1.000000000000000000, -1.373900992973642263E-15, -4.095874873834148624E-16 ) ) ;
#37599=VERTEX_POINT ( 'NONE', #27960 ) ;
#37610=DIRECTION ( 'NONE',  ( 1.000000000000000000, -1.373900992973642460E-15, -3.469446951953632924E-16 ) ) ;
#37623=LINE ( 'NONE', #21104, #22271 ) ;
#37638=ORIENTED_EDGE ( 'NONE', *, *, #22114, .T. ) ;
#37716=CARTESIAN_POINT ( 'NONE',  ( -126.0000000000000000, 1.230603612181083142E-13, -40.00000000000002842 ) ) ;
#37830=DIRECTION ( 'NONE',  ( -3.996523416598930318E-16, 2.658563593772947863E-15, 1.000000000000000000 ) ) ;
#37853=FACE_OUTER_BOUND ( 'NONE', #36568, .T. ) ;
#37871=COLOUR_RGB ( '', 0.31764706, 0.68627451, 0.89019608) ;
#37940=EDGE_LOOP ( 'NONE', ( #23677, #23494, #40034, #71 ) ) ;
#38081=CARTESIAN_POINT ( 'NONE',  ( 153.1499999999986414, 1.392576523351516607E-12, 9.999999999999959144 ) ) ;
#38086=ORIENTED_EDGE ( 'NONE', *, *, #38521, .T. ) ;
#38091=DIRECTION ( 'NONE',  ( 1.000000000000000000, -1.373900992973641277E-15, -5.551115123125812284E-16 ) ) ;
#38162=EDGE_CURVE ( 'NONE', #6244, #9154, #34895, .T. ) ;
#38259=CARTESIAN_POINT ( 'NONE',  ( -147.8499999999987438, -2.957510437470159335E-13, 10.00000000000004263 ) ) ;
#38278=VERTEX_POINT ( 'NONE', #15671 ) ;
#38290=EDGE_CURVE ( 'NONE', #13925, #23479, #20298, .T. ) ;
#38294=AXIS2_PLACEMENT_3D ( 'NONE', #20331, #16632, #3020 ) ;
#38365=ORIENTED_EDGE ( 'NONE', *, *, #11645, .F. ) ;
#38410=AXIS2_PLACEMENT_3D ( 'NONE', #18471, #37830, #41094 ) ;
#38437=DIRECTION ( 'NONE',  ( 1.000000000000000000, -1.373900992973641868E-15, -3.273063162220443081E-16 ) ) ;
#38456=AXIS2_PLACEMENT_3D ( 'NONE', #35392, #39501, #35588 ) ;
#38459=CARTESIAN_POINT ( 'NONE',  ( 1.598609366639573350E-14, -1.063425437509180407E-13, -40.00000000000000000 ) ) ;
#38481=ORIENTED_EDGE ( 'NONE', *, *, #38162, .T. ) ;
#38488=ORIENTED_EDGE ( 'NONE', *, *, #27740, .F. ) ;
#38521=EDGE_CURVE ( 'NONE', #27109, #23893, #28574, .T. ) ;
#38599=UNCERTAINTY_MEASURE_WITH_UNIT (LENGTH_MEASURE( 1.000000000000000082E-05 ), #18440, 'distance_accuracy_value', 'NONE');
#38635=CARTESIAN_POINT ( 'NONE',  ( 142.4999999999992895, -3.154162532185255727E-13, -45.00000000000004974 ) ) ;
#38669=AXIS2_PLACEMENT_3D ( 'NONE', #7277, #3120, #40220 ) ;
#38675=CARTESIAN_POINT ( 'NONE',  ( 139.5000000000000000, -2.144538195783117691E-13, 10.00000000000005684 ) ) ;
#38702=CIRCLE ( 'NONE', #25515, 2.649999999999957723 ) ;
#38744=ORIENTED_EDGE ( 'NONE', *, *, #39605, .T. ) ;
#38790=CYLINDRICAL_SURFACE ( 'NONE', #4044, 2.649999999999971934 ) ;
#38796=DIRECTION ( 'NONE',  ( 1.000000000000000000, 0.000000000000000000, -6.546126324440850663E-16 ) ) ;
#38808=EDGE_LOOP ( 'NONE', ( #23022, #23334, #6696, #16517 ) ) ;
#38885=SURFACE_STYLE_FILL_AREA ( #1373 ) ;
#38887=ORIENTED_EDGE ( 'NONE', *, *, #20013, .F. ) ;
#38905=FACE_OUTER_BOUND ( 'NONE', #41819, .T. ) ;
#38914=CIRCLE ( 'NONE', #7588, 2.649999999999971934 ) ;
#38916=ORIENTED_EDGE ( 'NONE', *, *, #33408, .F. ) ;
#38954=VERTEX_POINT ( 'NONE', #37716 ) ;
#38991=ADVANCED_FACE ( 'NONE', ( #12174 ), #32019, .T. ) ;
#39012=CARTESIAN_POINT ( 'NONE',  ( -2.797566391619251075E-15, 1.860994515641065082E-14, 7.000000000000002665 ) ) ;
#39024=ORIENTED_EDGE ( 'NONE', *, *, #9749, .T. ) ;
#39033=EDGE_CURVE ( 'NONE', #24964, #7188, #7004, .T. ) ;
#39097=ORIENTED_EDGE ( 'NONE', *, *, #928, .F. ) ;
#39098=DIRECTION ( 'NONE',  ( 1.000000000000000000, -1.373900992973642263E-15, -3.996523416598957436E-16 ) ) ;
#39118=ORIENTED_EDGE ( 'NONE', *, *, #39864, .T. ) ;
#39136=ORIENTED_EDGE ( 'NONE', *, *, #9767, .T. ) ;
#39217=ORIENTED_EDGE ( 'NONE', *, *, #28181, .T. ) ;
#39258=DIRECTION ( 'NONE',  ( 1.000000000000000000, -1.373900992973642263E-15, 0.000000000000000000 ) ) ;
#39344=CARTESIAN_POINT ( 'NONE',  ( -1.420922472151883646E-13, 9.833206111663764869E-13, 369.6955262170047831 ) ) ;
#39402=CARTESIAN_POINT ( 'NONE',  ( 1.798435537469519230E-14, -1.196353617197826191E-13, -44.99999999999999289 ) ) ;
#39429=CARTESIAN_POINT ( 'NONE',  ( 106.4195705685734623, 106.4195705685780524, 7.000000000000250466 ) ) ;
#39430=CIRCLE ( 'NONE', #35238, 1.999999999999988010 ) ;
#39431=PLANE ( 'NONE',  #16813 ) ;
#39446=CARTESIAN_POINT ( 'NONE',  ( 1.039096088315723056E-14, -6.912265343809663812E-14, -26.00000000000000355 ) ) ;
#39501=DIRECTION ( 'NONE',  ( -3.996523416598930318E-16, 2.658563593772947863E-15, 1.000000000000000000 ) ) ;
#39534=DIRECTION ( 'NONE',  ( 1.000000000000000000, 0.000000000000000000, -3.273063162220425331E-16 ) ) ;
#39554=CIRCLE ( 'NONE', #29818, 2.649999999999973266 ) ;
#39605=EDGE_CURVE ( 'NONE', #24835, #38278, #34923, .T. ) ;
#39645=DIRECTION ( 'NONE',  ( 1.000000000000000000, -1.373900992973642263E-15, -3.996523416598957436E-16 ) ) ;
#39737=EDGE_LOOP ( 'NONE', ( #11738, #1351 ) ) ;
#39814=FACE_OUTER_BOUND ( 'NONE', #20997, .T. ) ;
#39852=ORIENTED_EDGE ( 'NONE', *, *, #12745, .F. ) ;
#39864=EDGE_CURVE ( 'NONE', #19368, #28359, #41914, .T. ) ;
#39865=EDGE_LOOP ( 'NONE', ( #22568, #7134 ) ) ;
#39874=VERTEX_POINT ( 'NONE', #7695 ) ;
#39950=CARTESIAN_POINT ( 'NONE',  ( -106.4195705685741871, -106.4195705685773135, 6.999999999999754863 ) ) ;
#39994=ORIENTED_EDGE ( 'NONE', *, *, #9767, .F. ) ;
#40034=ORIENTED_EDGE ( 'NONE', *, *, #37465, .T. ) ;
#40067=APPLICATION_CONTEXT ( 'automotive_design' ) ;
#40139=EDGE_CURVE ( 'NONE', #43139, #29204, #18995, .T. ) ;
#40157=CIRCLE ( 'NONE', #17340, 2.649999999999979039 ) ;
#40189=CARTESIAN_POINT ( 'NONE',  ( 1.598609366639573350E-14, -1.063425437509180407E-13, -40.00000000000000000 ) ) ;
#40196=ADVANCED_FACE ( 'NONE', ( #33188 ), #33612, .F. ) ;
#40216=CIRCLE ( 'NONE', #3264, 125.9999999999993605 ) ;
#40220=DIRECTION ( 'NONE',  ( 1.000000000000000000, -1.373900992973642263E-15, -3.016910393003158636E-16 ) ) ;
#40235=CARTESIAN_POINT ( 'NONE',  ( -153.1499999999986699, -2.921326824731409465E-13, 7.000000000000041744 ) ) ;
#40256=LINE ( 'NONE', #10387, #9873 ) ;
#40291=ORIENTED_EDGE ( 'NONE', *, *, #2638, .T. ) ;
#40367=EDGE_CURVE ( 'NONE', #19368, #29604, #34699, .T. ) ;
#40376=CARTESIAN_POINT ( 'NONE',  ( -150.4999999999986926, -2.921102061156358310E-13, 10.00000000000004441 ) ) ;
#40383=ORIENTED_EDGE ( 'NONE', *, *, #14270, .F. ) ;
#40491=ADVANCED_FACE ( 'NONE', ( #22293 ), #28815, .T. ) ;
#40514=CYLINDRICAL_SURFACE ( 'NONE', #42072, 125.9999999999993605 ) ;
#40522=DIRECTION ( 'NONE',  ( 1.000000000000000000, -1.373900992973642460E-15, -3.469446951953632924E-16 ) ) ;
#40594=CARTESIAN_POINT ( 'NONE',  ( -130.0000000000000000, 1.285559651900026877E-13, -40.00000000000004974 ) ) ;
#40628=MECHANICAL_DESIGN_GEOMETRIC_PRESENTATION_REPRESENTATION('',(#6505),#33701);
#40840=AXIS2_PLACEMENT_3D ( 'NONE', #5921, #5714, #15568 ) ;
#40842=DIRECTION ( 'NONE',  ( 1.000000000000000000, -1.373900992973641277E-15, -5.551115123125812284E-16 ) ) ;
#40851=DIRECTION ( 'NONE',  ( 3.996523416598930318E-16, -2.658563593772947863E-15, -1.000000000000000000 ) ) ;
#40863=CIRCLE ( 'NONE', #22120, 2.649999999999973266 ) ;
#40889=ORIENTED_EDGE ( 'NONE', *, *, #35908, .F. ) ;
#40947=VERTEX_POINT ( 'NONE', #28122 ) ;
#41054=ORIENTED_EDGE ( 'NONE', *, *, #33861, .T. ) ;
#41078=EDGE_LOOP ( 'NONE', ( #35911, #7301 ) ) ;
#41083=DIRECTION ( 'NONE',  ( 3.996523416598993920E-16, 2.658563593772947074E-15, 1.000000000000000000 ) ) ;
#41094=DIRECTION ( 'NONE',  ( 1.000000000000000000, 0.000000000000000000, -6.546126324440850663E-16 ) ) ;
#41099=FACE_OUTER_BOUND ( 'NONE', #11680, .T. ) ;
#41129=AXIS2_PLACEMENT_3D ( 'NONE', #28109, #35056, #41374 ) ;
#41130=AXIS2_PLACEMENT_3D ( 'NONE', #7692, #21271, #40842 ) ;
#41153=CARTESIAN_POINT ( 'NONE',  ( -158.5000000000000284, 2.597717496998779451E-13, 9.999999999999937828 ) ) ;
#41159=CARTESIAN_POINT ( 'NONE',  ( -142.4999999999992326, 9.359674666681006779E-14, -44.99999999999993605 ) ) ;
#41176=CARTESIAN_POINT ( 'NONE',  ( -2.649999999999784528, -150.5000000000013642, 9.999999999999586109 ) ) ;
#41243=ORIENTED_EDGE ( 'NONE', *, *, #21246, .T. ) ;
#41329=CARTESIAN_POINT ( 'NONE',  ( 104.9999999999993321, -2.293336392629658115E-13, -32.00000000000000000 ) ) ;
#41336=DIRECTION ( 'NONE',  ( -3.996523416598930318E-16, 2.658563593772947863E-15, 1.000000000000000000 ) ) ;
#41359=FACE_OUTER_BOUND ( 'NONE', #36242, .T. ) ;
#41365=AXIS2_PLACEMENT_3D ( 'NONE', #10752, #4180, #34094 ) ;
#41374=DIRECTION ( 'NONE',  ( 1.000000000000000000, 0.000000000000000000, -3.273063162220425331E-16 ) ) ;
#41417=CARTESIAN_POINT ( 'NONE',  ( -3.996523416598931009E-15, 2.658563593772952281E-14, 10.00000000000000178 ) ) ;
#41480=ADVANCED_FACE ( 'NONE', ( #32127 ), #2636, .T. ) ;
#41484=VERTEX_POINT ( 'NONE', #42766 ) ;
#41503=AXIS2_PLACEMENT_3D ( 'NONE', #23268, #17538, #888 ) ;
#41507=FILL_AREA_STYLE_COLOUR ( '', #37871 ) ;
#41554=DIRECTION ( 'NONE',  ( -3.996523416598930318E-16, 2.658563593772947863E-15, 1.000000000000000000 ) ) ;
#41588=VECTOR ( 'NONE', #24134, 1000.000000000000000 ) ;
#41600=VECTOR ( 'NONE', #20662, 1000.000000000000000 ) ;
#41746=CARTESIAN_POINT ( 'NONE',  ( -2.797566391619251075E-15, 1.860994515641065082E-14, 7.000000000000002665 ) ) ;
#41819=EDGE_LOOP ( 'NONE', ( #17671, #18976 ) ) ;
#41858=CYLINDRICAL_SURFACE ( 'NONE', #33460, 139.4999999999992610 ) ;
#41861=DIRECTION ( 'NONE',  ( 3.996523416598930318E-16, -2.658563593772947863E-15, -1.000000000000000000 ) ) ;
#41878=EDGE_LOOP ( 'NONE', ( #2396, #22664 ) ) ;
#41909=EDGE_LOOP ( 'NONE', ( #38365, #33565 ) ) ;
#41914=CIRCLE ( 'NONE', #22444, 2.649999999999957723 ) ;
#41917=CARTESIAN_POINT ( 'NONE',  ( 4.858130855304160865E-15, 5.778671572660278980E-15, 2.000000000000001776 ) ) ;
#41935=( NAMED_UNIT ( * ) PLANE_ANGLE_UNIT ( ) SI_UNIT ( $, .RADIAN. ) );
#42038=CARTESIAN_POINT ( 'NONE',  ( 12.49999999999995026, -1.235163061630884815E-13, -40.00000000000000711 ) ) ;
#42072=AXIS2_PLACEMENT_3D ( 'NONE', #33554, #17451, #21158 ) ;
#42083=AXIS2_PLACEMENT_3D ( 'NONE', #41746, #41083, #11888 ) ;
#42096=EDGE_LOOP ( 'NONE', ( #9359, #13492 ) ) ;
#42139=( LENGTH_UNIT ( ) NAMED_UNIT ( * ) SI_UNIT ( .MILLI., .METRE. ) );
#42151=DIRECTION ( 'NONE',  ( 1.000000000000000000, -1.373900992973642263E-15, -3.996523416598957436E-16 ) ) ;
#42175=CIRCLE ( 'NONE', #35218, 142.4999999999992610 ) ;
#42217=ORIENTED_EDGE ( 'NONE', *, *, #1513, .F. ) ;
#42222=ORIENTED_EDGE ( 'NONE', *, *, #2057, .T. ) ;
#42250=AXIS2_PLACEMENT_3D ( 'NONE', #26602, #32702, #36178 ) ;
#42262=DIRECTION ( 'NONE',  ( 1.000000000000000000, -1.373900992973642066E-15, -3.979293995072266947E-16 ) ) ;
#42334=FACE_OUTER_BOUND ( 'NONE', #14389, .T. ) ;
#42363=FILL_AREA_STYLE ('',( #41507 ) ) ;
#42388=DIRECTION ( 'NONE',  ( -0.2140725878556618000, 0.9768177553304300265, 2.796485154102059642E-15 ) ) ;
#42401=VERTEX_POINT ( 'NONE', #42038 ) ;
#42478=DIRECTION ( 'NONE',  ( 3.996523416598930318E-16, -2.658563593772947863E-15, -1.000000000000000000 ) ) ;
#42550=ORIENTED_EDGE ( 'NONE', *, *, #14270, .T. ) ;
#42586=DIRECTION ( 'NONE',  ( 1.000000000000000000, -1.373900992973641868E-15, -4.049512215214018063E-16 ) ) ;
#42660=UNCERTAINTY_MEASURE_WITH_UNIT (LENGTH_MEASURE( 1.000000000000000082E-05 ), #42139, 'distance_accuracy_value', 'NONE');
#42679=VECTOR ( 'NONE', #34424, 1000.000000000000000 ) ;
#42766=CARTESIAN_POINT ( 'NONE',  ( -130.0000000000000000, 1.285559651900030663E-13, 1.999999999999930278 ) ) ;
#42772=AXIS2_PLACEMENT_3D ( 'NONE', #23640, #30160, #215 ) ;
#42787=CARTESIAN_POINT ( 'NONE',  ( 1.039096088315723056E-14, -6.912265343809663812E-14, -26.00000000000000355 ) ) ;
#42798=ORIENTED_EDGE ( 'NONE', *, *, #10056, .F. ) ;
#42812=DIRECTION ( 'NONE',  ( -1.000000000000000000, 1.373900992973641868E-15, 3.469446951953632924E-16 ) ) ;
#42822=ORIENTED_EDGE ( 'NONE', *, *, #33624, .F. ) ;
#42867=CARTESIAN_POINT ( 'NONE',  ( -2.649999999999776090, -150.5000000000013642, 9.999999999999587885 ) ) ;
#42873=CARTESIAN_POINT ( 'NONE',  ( 2.650000000000181988, -150.5000000000013642, 9.999999999999584332 ) ) ;
#42885=AXIS2_PLACEMENT_3D ( 'NONE', #14383, #37483, #1470 ) ;
#42902=DIRECTION ( 'NONE',  ( 3.996523416598930318E-16, -2.658563593772947863E-15, -1.000000000000000000 ) ) ;
#42929=CARTESIAN_POINT ( 'NONE',  ( -139.5000000000000000, 1.517807346132285267E-13, 9.999999999999946709 ) ) ;
#42975=VERTEX_POINT ( 'NONE', #4368 ) ;
#43006=CARTESIAN_POINT ( 'NONE',  ( -22.99999999999998579, -5.613287575611360052E-14, -26.00000000000001421 ) ) ;
#43039=FACE_BOUND ( 'NONE', #28228, .T. ) ;
#43084=LINE ( 'NONE', #33696, #41588 ) ;
#43091=ORIENTED_EDGE ( 'NONE', *, *, #18569, .T. ) ;
#43115=DIRECTION ( 'NONE',  ( 1.000000000000000000, -1.373900992973641671E-15, -3.895519384649692070E-16 ) ) ;
#43139=VERTEX_POINT ( 'NONE', #27902 ) ;
#43164=CARTESIAN_POINT ( 'NONE',  ( 2.650000000000182876, -150.5000000000013642, 6.999999999999585221 ) ) ;
#43171=ADVANCED_FACE ( 'NONE', ( #34199 ), #40514, .F. ) ;
#43176=DIRECTION ( 'NONE',  ( 3.996523416598930318E-16, -2.658563593772947863E-15, -1.000000000000000000 ) ) ;
ENDSEC;
END-ISO-10303-21;
